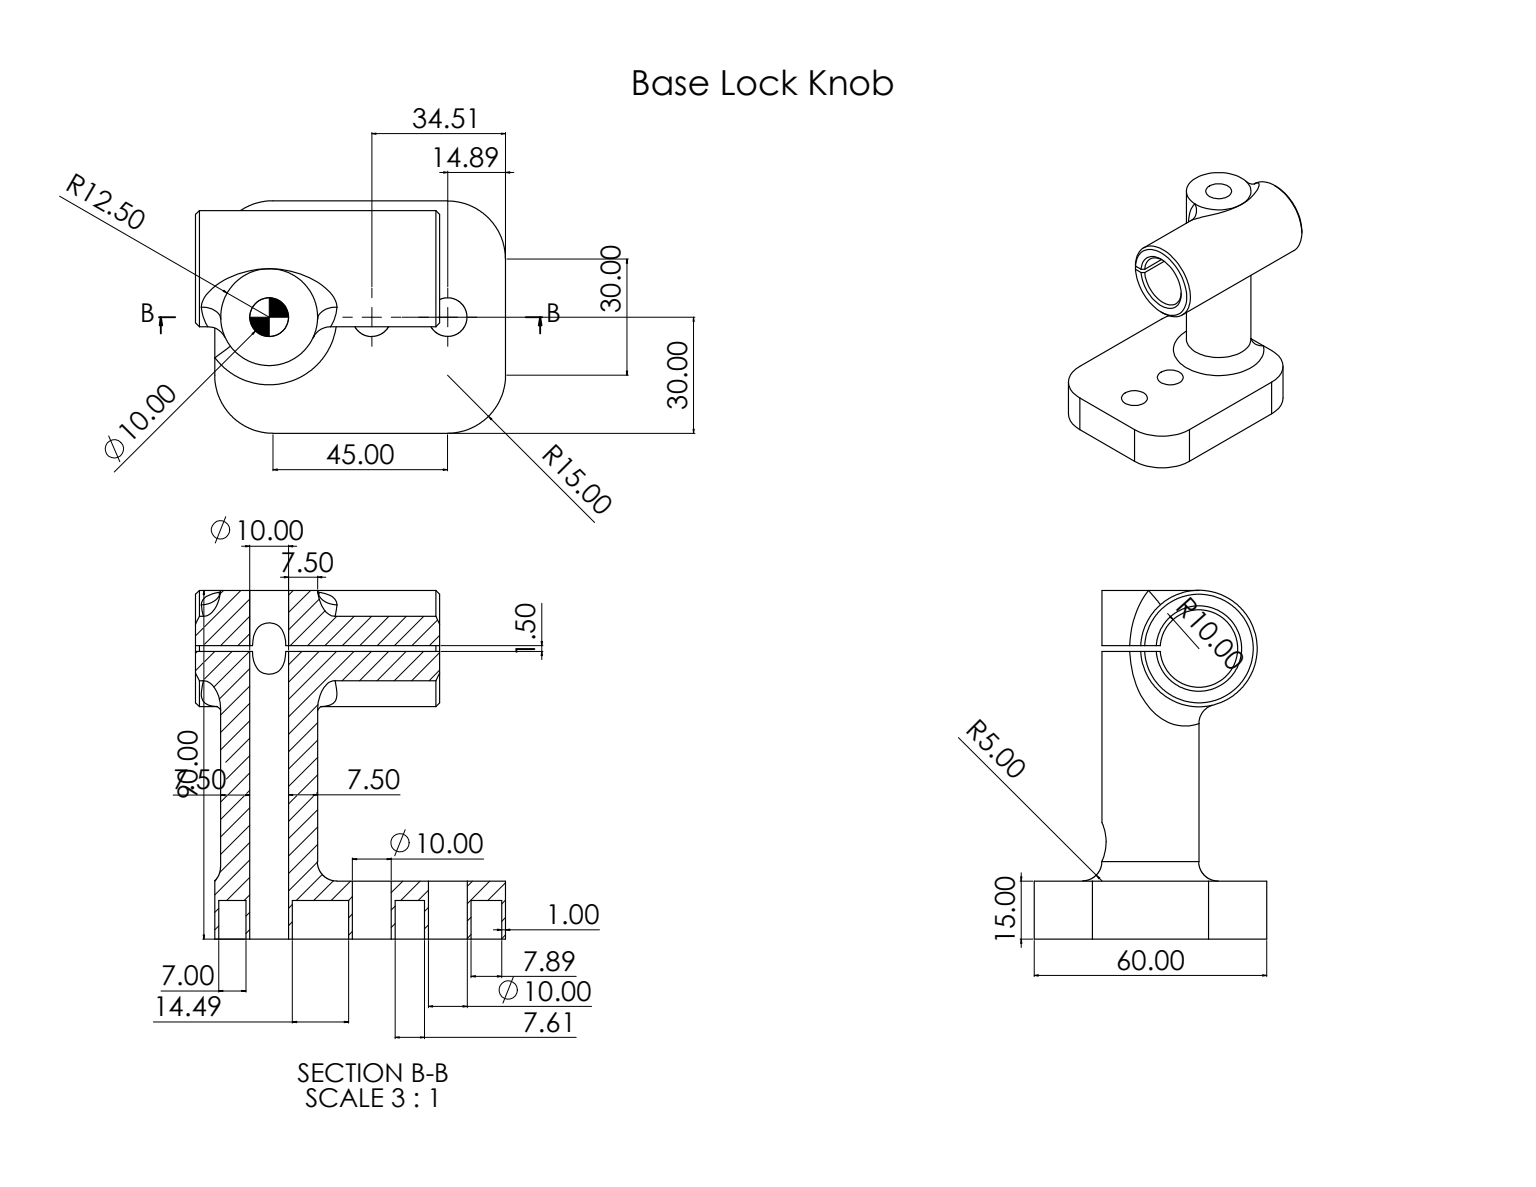
ISO-10303-21;
HEADER;
FILE_DESCRIPTION (('STEP AP214'),
    '1' );
FILE_NAME ('Base Lock Knob.step',
    '2026-10-26T22:46:44',
    ( '' ),
    ( '' ),
    'SwSTEP 2.0',
    'SolidWorks 2025',
    '' );
FILE_SCHEMA (( 'AUTOMOTIVE_DESIGN' ));
ENDSEC;

DATA;
#13=EDGE_CURVE ( 'NONE', #4124, #14697, #820, .T. ) ;
#15=CARTESIAN_POINT ( 'NONE',  ( -25.96080279087190945, 79.85293219504170281, -10.39653350028737755 ) ) ;
#19=CARTESIAN_POINT ( 'NONE',  ( 0.000000000000000000, -10.00000000000000000, 0.000000000000000000 ) ) ;
#40=CARTESIAN_POINT ( 'NONE',  ( -32.23733050826358237, 69.70612202061964524, 1.777571403100950187 ) ) ;
#44=CARTESIAN_POINT ( 'NONE',  ( -28.41953442586123302, 80.00000000005270806, -1.424835221693572684 ) ) ;
#49=AXIS2_PLACEMENT_3D ( 'NONE', #5119, #19642, #8405 ) ;
#53=ORIENTED_EDGE ( 'NONE', *, *, #309, .F. ) ;
#62=LINE ( 'NONE', #1856, #5490 ) ;
#65=CIRCLE ( 'NONE', #5111, 12.50000000000000000 ) ;
#69=CARTESIAN_POINT ( 'NONE',  ( -27.55705705607979894, 6.378909713838078588, -4.810857297669037358 ) ) ;
#72=ADVANCED_FACE ( 'NONE', ( #4104, #6856 ), #20110, .T. ) ;
#74=CARTESIAN_POINT ( 'NONE',  ( -3.712242387446013758, 47.26449505096422854, -2.316332963494041497 ) ) ;
#75=AXIS2_PLACEMENT_3D ( 'NONE', #8179, #20707, #4902 ) ;
#78=CARTESIAN_POINT ( 'NONE',  ( -4.898149591010308335, 50.01850704181430984, -13.27720951148779349 ) ) ;
#82=EDGE_CURVE ( 'NONE', #14650, #1521, #9980, .T. ) ;
#90=FACE_OUTER_BOUND ( 'NONE', #11303, .T. ) ;
#94=CARTESIAN_POINT ( 'NONE',  ( -20.20766917169448007, 62.83385617594171180, -2.712160011935111914 ) ) ;
#97=CARTESIAN_POINT ( 'NONE',  ( -14.59739189792666281, 58.60404727593866170, -4.812026853405405369 ) ) ;
#107=CARTESIAN_POINT ( 'NONE',  ( -32.72405129661866141, 57.94895811088655080, 0.7443064298479508123 ) ) ;
#126=CARTESIAN_POINT ( 'NONE',  ( -0.1767699604045824824, 64.25000000000000000, 2.481238266578627449 ) ) ;
#133=DIRECTION ( 'NONE',  ( -0.000000000000000000, 1.000000000000000000, -0.000000000000000000 ) ) ;
#143=CARTESIAN_POINT ( 'NONE',  ( -31.87136685185827645, 66.76123571212177410, 2.404802591979305237 ) ) ;
#151=CARTESIAN_POINT ( 'NONE',  ( -28.39898833977742854, 64.25000000000000000, 3.829121630900767848 ) ) ;
#162=EDGE_CURVE ( 'NONE', #4703, #13744, #13389, .T. ) ;
#166=VERTEX_POINT ( 'NONE', #7371 ) ;
#168=CARTESIAN_POINT ( 'NONE',  ( -15.61408887313298166, 45.63508326896292289, -12.50000000000000533 ) ) ;
#173=CARTESIAN_POINT ( 'NONE',  ( 0.8637328751229490509, 57.32143202600091314, 0.4056442452730588677 ) ) ;
#174=CARTESIAN_POINT ( 'NONE',  ( 0.2936549083987780584, 78.35468191082874512, -5.667085693055155637 ) ) ;
#180=ORIENTED_EDGE ( 'NONE', *, *, #8626, .T. ) ;
#196=VECTOR ( 'NONE', #4579, 1000.000000000000000 ) ;
#201=CARTESIAN_POINT ( 'NONE',  ( -32.31535884961043337, 59.90787884595005863, 1.627344972937480483 ) ) ;
#223=CYLINDRICAL_SURFACE ( 'NONE', #8286, 5.000000000000000000 ) ;
#228=EDGE_LOOP ( 'NONE', ( #1966, #14551, #9394, #914, #2067, #12471, #14821, #17580, #5403, #1919 ) ) ;
#245=VERTEX_POINT ( 'NONE', #13977 ) ;
#253=AXIS2_PLACEMENT_3D ( 'NONE', #1126, #2508, #8850 ) ;
#262=VECTOR ( 'NONE', #1217, 1000.000000000000000 ) ;
#269=CARTESIAN_POINT ( 'NONE',  ( -4.599716269004222369, 61.16723911170964811, 5.137000474222295665 ) ) ;
#273=CARTESIAN_POINT ( 'NONE',  ( 1.235636163673195176, 55.55531401624686794, -0.8411524222362073422 ) ) ;
#274=CARTESIAN_POINT ( 'NONE',  ( -27.29860958162435480, 65.74999999999997158, 5.347094680480812379 ) ) ;
#278=CARTESIAN_POINT ( 'NONE',  ( -28.99999999999999289, 0.000000000000000000, 15.00000000000000178 ) ) ;
#285=FACE_OUTER_BOUND ( 'NONE', #6570, .T. ) ;
#287=EDGE_LOOP ( 'NONE', ( #14816, #1290 ) ) ;
#301=CARTESIAN_POINT ( 'NONE',  ( -33.51155206502836137, 53.04833639938227208, -3.407080289749979229 ) ) ;
#309=EDGE_CURVE ( 'NONE', #20070, #6727, #13759, .T. ) ;
#324=EDGE_CURVE ( 'NONE', #1328, #16503, #11374, .T. ) ;
#329=AXIS2_PLACEMENT_3D ( 'NONE', #7780, #14388, #14489 ) ;
#336=PLANE ( 'NONE',  #16281 ) ;
#345=ORIENTED_EDGE ( 'NONE', *, *, #6765, .T. ) ;
#347=ORIENTED_EDGE ( 'NONE', *, *, #464, .T. ) ;
#348=ADVANCED_FACE ( 'NONE', ( #1860 ), #11088, .F. ) ;
#353=ORIENTED_EDGE ( 'NONE', *, *, #18968, .F. ) ;
#355=CARTESIAN_POINT ( 'NONE',  ( -21.06087829250213161, 79.98244021547201044, -11.72107194671396790 ) ) ;
#358=EDGE_CURVE ( 'NONE', #6609, #4749, #6287, .T. ) ;
#368=DIRECTION ( 'NONE',  ( -0.000000000000000000, -1.000000000000000000, -0.000000000000000000 ) ) ;
#369=EDGE_CURVE ( 'NONE', #14650, #14697, #6503, .T. ) ;
#372=FACE_OUTER_BOUND ( 'NONE', #9443, .T. ) ;
#373=CARTESIAN_POINT ( 'NONE',  ( -4.811817756148304426, 79.75568800831774752, -9.793444445058595349 ) ) ;
#387=CARTESIAN_POINT ( 'NONE',  ( -3.556084784758247075, 50.96167829366792290, 1.269699694002965007 ) ) ;
#388=CARTESIAN_POINT ( 'NONE',  ( -9.537558382401318369, 79.97813440949151698, -11.66361662172994507 ) ) ;
#396=ORIENTED_EDGE ( 'NONE', *, *, #17876, .T. ) ;
#407=CIRCLE ( 'NONE', #12256, 5.999999999999989342 ) ;
#408=DIRECTION ( 'NONE',  ( -1.000000000000000000, 0.000000000000000000, 0.000000000000000000 ) ) ;
#409=CARTESIAN_POINT ( 'NONE',  ( -15.99999999999999289, 80.00000000000000000, 0.000000000000000000 ) ) ;
#417=CARTESIAN_POINT ( 'NONE',  ( -33.37417213237042546, 54.75746433087826404, -1.535552296325748189 ) ) ;
#422=EDGE_CURVE ( 'NONE', #16527, #15321, #7895, .T. ) ;
#434=( BOUNDED_CURVE ( )  B_SPLINE_CURVE ( 3, ( #6259, #9555, #12753, #12546 ),
 .UNSPECIFIED., .F., .T. ) 
 B_SPLINE_CURVE_WITH_KNOTS ( ( 4, 4 ),
 ( 4.913746901175024107, 6.283185307179586232 ),
 .UNSPECIFIED. ) 
 CURVE ( )  GEOMETRIC_REPRESENTATION_ITEM ( )  RATIONAL_B_SPLINE_CURVE ( ( 1.000000000000000000, 0.8497311128276563430, 0.8497311128276563430, 1.000000000000000000 ) ) 
 REPRESENTATION_ITEM ( '' )  );
#448=ORIENTED_EDGE ( 'NONE', *, *, #2524, .T. ) ;
#461=CARTESIAN_POINT ( 'NONE',  ( -17.30116400286886247, 79.99994664032418257, -12.45114708371502665 ) ) ;
#463=CARTESIAN_POINT ( 'NONE',  ( 30.00000000000000355, 5.000000000000000000, 30.00000000000000000 ) ) ;
#464=EDGE_CURVE ( 'NONE', #15321, #2307, #18152, .T. ) ;
#476=CARTESIAN_POINT ( 'NONE',  ( -0.1767699604045824824, 64.25000000000000000, 2.481238266578627449 ) ) ;
#477=CARTESIAN_POINT ( 'NONE',  ( -3.836698435374707561, 79.99999999983937471, -2.903060217168568435 ) ) ;
#482=LINE ( 'NONE', #19857, #18341 ) ;
#487=CARTESIAN_POINT ( 'NONE',  ( -26.66796757275972851, 5.894401750582999533, 6.542839447999508451 ) ) ;
#491=VERTEX_POINT ( 'NONE', #4071 ) ;
#493=CARTESIAN_POINT ( 'NONE',  ( -3.931445803941664430, 46.62695496839331355, -3.273709564003291383 ) ) ;
#496=CARTESIAN_POINT ( 'NONE',  ( 0.5172280101801079999, 58.91385993483535799, 1.214474307743183434 ) ) ;
#497=CARTESIAN_POINT ( 'NONE',  ( 0.4210663660453498047, 78.26446952993892126, -5.493235020936472424 ) ) ;
#501=DIRECTION ( 'NONE',  ( -0.000000000000000000, -1.000000000000000000, -0.000000000000000000 ) ) ;
#520=CARTESIAN_POINT ( 'NONE',  ( -32.92944801084382078, 57.01857061577523922, 0.2052755498065614581 ) ) ;
#532=DIRECTION ( 'NONE',  ( -0.000000000000000000, 1.000000000000000000, -0.000000000000000000 ) ) ;
#533=AXIS2_PLACEMENT_3D ( 'NONE', #6159, #10536, #10317 ) ;
#541=CARTESIAN_POINT ( 'NONE',  ( 30.10683012259193703, 0.000000000000000000, 0.000000000000000000 ) ) ;
#553=( BOUNDED_CURVE ( )  B_SPLINE_CURVE ( 3, ( #9239, #19121, #12236, #18698 ),
 .UNSPECIFIED., .F., .F. ) 
 B_SPLINE_CURVE_WITH_KNOTS ( ( 4, 4 ),
 ( 0.000000000000000000, 1.369438406004562347 ),
 .UNSPECIFIED. ) 
 CURVE ( )  GEOMETRIC_REPRESENTATION_ITEM ( )  RATIONAL_B_SPLINE_CURVE ( ( 1.000000000000000000, 0.8497311128276563430, 0.8497311128276563430, 1.000000000000000000 ) ) 
 REPRESENTATION_ITEM ( '' )  );
#554=ORIENTED_EDGE ( 'NONE', *, *, #4724, .T. ) ;
#563=CARTESIAN_POINT ( 'NONE',  ( -26.10629707152433809, 79.63451458383349291, -9.058872303758411348 ) ) ;
#569=CARTESIAN_POINT ( 'NONE',  ( -30.20545447418457385, 64.25000000000001421, 2.744335235139487406 ) ) ;
#575=CARTESIAN_POINT ( 'NONE',  ( -2.600405991085453561, 77.88264414865945184, -4.670285688179051320 ) ) ;
#577=ORIENTED_EDGE ( 'NONE', *, *, #4172, .T. ) ;
#580=DIRECTION ( 'NONE',  ( 1.000000000000000000, 0.000000000000000000, 0.000000000000000000 ) ) ;
#583=EDGE_CURVE ( 'NONE', #14019, #631, #10846, .T. ) ;
#585=CARTESIAN_POINT ( 'NONE',  ( -29.99999999999999645, 5.000000000000000000, 9.729160503328165177 ) ) ;
#595=CARTESIAN_POINT ( 'NONE',  ( -3.729411824114762020, 52.78418889159976857, -3.786816875109808578 ) ) ;
#598=DIRECTION ( 'NONE',  ( -1.000000000000000000, -0.000000000000000000, -0.000000000000000000 ) ) ;
#603=CARTESIAN_POINT ( 'NONE',  ( 27.66662763442663220, 64.25000000000000000, -1.859747928060467181 ) ) ;
#615=CARTESIAN_POINT ( 'NONE',  ( -19.02430517209115735, 70.26110273505831572, -3.991204510516646931 ) ) ;
#616=EDGE_CURVE ( 'NONE', #631, #3306, #11174, .T. ) ;
#618=EDGE_CURVE ( 'NONE', #9039, #9755, #2936, .T. ) ;
#621=CARTESIAN_POINT ( 'NONE',  ( -28.23075158081314484, 53.16826294859335889, 2.609184450367471708 ) ) ;
#626=ORIENTED_EDGE ( 'NONE', *, *, #616, .T. ) ;
#631=VERTEX_POINT ( 'NONE', #3318 ) ;
#639=CARTESIAN_POINT ( 'NONE',  ( 30.00000000000000355, 5.000000000000000000, -15.00000000000000000 ) ) ;
#653=ORIENTED_EDGE ( 'NONE', *, *, #12072, .F. ) ;
#655=CARTESIAN_POINT ( 'NONE',  ( -14.99999999999999645, 0.000000000000000000, -15.00000000000000000 ) ) ;
#659=EDGE_LOOP ( 'NONE', ( #1271, #18731 ) ) ;
#661=CARTESIAN_POINT ( 'NONE',  ( -17.30014261508840434, 80.00000000000054001, -12.43489149392628512 ) ) ;
#662=FACE_OUTER_BOUND ( 'NONE', #2324, .T. ) ;
#664=ORIENTED_EDGE ( 'NONE', *, *, #14243, .F. ) ;
#675=EDGE_CURVE ( 'NONE', #11638, #6609, #8654, .T. ) ;
#681=VERTEX_POINT ( 'NONE', #19127 ) ;
#682=DIRECTION ( 'NONE',  ( -0.000000000000000000, 1.000000000000000000, -0.000000000000000000 ) ) ;
#686=DIRECTION ( 'NONE',  ( -1.000000000000000000, -0.000000000000000000, -0.000000000000000000 ) ) ;
#693=VECTOR ( 'NONE', #17106, 1000.000000000000000 ) ;
#702=EDGE_CURVE ( 'NONE', #19907, #9631, #6632, .T. ) ;
#710=CIRCLE ( 'NONE', #14277, 13.99999999999999822 ) ;
#711=EDGE_LOOP ( 'NONE', ( #17334, #865, #11449, #20358 ) ) ;
#714=CARTESIAN_POINT ( 'NONE',  ( 30.00000000000000355, 0.000000000000000000, -15.00000000000000000 ) ) ;
#720=DIRECTION ( 'NONE',  ( 0.000000000000000000, 0.000000000000000000, -1.000000000000000000 ) ) ;
#725=CYLINDRICAL_SURFACE ( 'NONE', #12270, 12.50000000000000000 ) ;
#726=CARTESIAN_POINT ( 'NONE',  ( -15.04600911323590218, 50.47255456144257835, -16.23554317993713170 ) ) ;
#737=ORIENTED_EDGE ( 'NONE', *, *, #2963, .F. ) ;
#739=DIRECTION ( 'NONE',  ( -0.000000000000000000, -0.000000000000000000, 1.000000000000000000 ) ) ;
#745=ORIENTED_EDGE ( 'NONE', *, *, #358, .F. ) ;
#752=DIRECTION ( 'NONE',  ( 0.000000000000000000, -0.000000000000000000, -1.000000000000000000 ) ) ;
#753=FACE_OUTER_BOUND ( 'NONE', #17256, .T. ) ;
#774=CARTESIAN_POINT ( 'NONE',  ( -16.26047902139016088, 79.99999999999998579, -12.49895143242785522 ) ) ;
#776=CARTESIAN_POINT ( 'NONE',  ( 30.00000000000000355, -10.00000000000000000, -28.99999999999999645 ) ) ;
#788=CARTESIAN_POINT ( 'NONE',  ( -15.47785876946503691, 80.00000332749893062, -12.49385289755957729 ) ) ;
#796=CARTESIAN_POINT ( 'NONE',  ( -28.50008649836227193, 6.470284334177582863, 0.3892821999670322275 ) ) ;
#801=AXIS2_PLACEMENT_3D ( 'NONE', #9097, #5597, #15294 ) ;
#810=ORIENTED_EDGE ( 'NONE', *, *, #11877, .F. ) ;
#819=CIRCLE ( 'NONE', #15126, 14.99999999999999645 ) ;
#820=LINE ( 'NONE', #20002, #17114 ) ;
#825=CARTESIAN_POINT ( 'NONE',  ( -10.99999999999999822, 15.09941697557068530, 0.9999999999999991118 ) ) ;
#826=DIRECTION ( 'NONE',  ( -0.000000000000000000, -0.000000000000000000, 1.000000000000000000 ) ) ;
#827=CARTESIAN_POINT ( 'NONE',  ( -17.49467092514650801, 49.50700362264424115, -12.43228238208896030 ) ) ;
#829=VECTOR ( 'NONE', #16903, 1000.000000000000000 ) ;
#851=CARTESIAN_POINT ( 'NONE',  ( -13.77465266732642846, 19.58876728727312511, 12.30409294039043466 ) ) ;
#854=CARTESIAN_POINT ( 'NONE',  ( -28.16307471351787228, 76.23982303504115521, 2.898234736985794591 ) ) ;
#865=ORIENTED_EDGE ( 'NONE', *, *, #17437, .F. ) ;
#868=EDGE_CURVE ( 'NONE', #1492, #2398, #16138, .T. ) ;
#876=CARTESIAN_POINT ( 'NONE',  ( -11.09376813494104397, 14.43059931244999028, 0.9644707416441876680 ) ) ;
#889=CARTESIAN_POINT ( 'NONE',  ( 30.10683012259193703, -24.14213562373095456, 0.000000000000000000 ) ) ;
#890=CARTESIAN_POINT ( 'NONE',  ( -15.47785959468120431, 80.00000000000014211, -12.49180211257053230 ) ) ;
#894=AXIS2_PLACEMENT_3D ( 'NONE', #1472, #17166, #19175 ) ;
#895=CARTESIAN_POINT ( 'NONE',  ( -12.69376962344485449, 11.33472108774821763, 12.05717403569970969 ) ) ;
#900=CARTESIAN_POINT ( 'NONE',  ( -28.22855330669906593, 8.912322265355541617, 2.677539729764461196 ) ) ;
#907=TOROIDAL_SURFACE ( 'NONE', #12088, 17.50000000000000000, 5.000000000000000000 ) ;
#914=ORIENTED_EDGE ( 'NONE', *, *, #14759, .T. ) ;
#916=LINE ( 'NONE', #12659, #16572 ) ;
#919=EDGE_CURVE ( 'NONE', #2330, #10554, #16387, .T. ) ;
#932=CARTESIAN_POINT ( 'NONE',  ( -14.62719308666609486, 45.60972712416246111, -12.42922832581293413 ) ) ;
#947=PLANE ( 'NONE',  #10845 ) ;
#948=CARTESIAN_POINT ( 'NONE',  ( -1.752364627967215149, 50.08700668601604633, -10.77852995906744304 ) ) ;
#949=LINE ( 'NONE', #17067, #3578 ) ;
#993=CARTESIAN_POINT ( 'NONE',  ( -4.579930894573177369, 68.94695149080686747, 5.083831496961729535 ) ) ;
#1002=CARTESIAN_POINT ( 'NONE',  ( -15.66959223257168432, 10.09941697557068707, 12.50000000000000000 ) ) ;
#1005=CARTESIAN_POINT ( 'NONE',  ( -26.38519111739858758, 79.82398913006802843, -10.19891841068203142 ) ) ;
#1007=CARTESIAN_POINT ( 'NONE',  ( -33.99999999999997868, 64.25000000000000000, -2.528164662410438357 ) ) ;
#1022=ORIENTED_EDGE ( 'NONE', *, *, #6255, .F. ) ;
#1034=AXIS2_PLACEMENT_3D ( 'NONE', #19639, #3534, #16472 ) ;
#1035=LINE ( 'NONE', #20422, #19941 ) ;
#1038=CARTESIAN_POINT ( 'NONE',  ( -13.06364034290321463, 49.50854601617997020, -12.17427138426762312 ) ) ;
#1050=VECTOR ( 'NONE', #11952, 1000.000000000000000 ) ;
#1054=CARTESIAN_POINT ( 'NONE',  ( -15.99999999999999289, 64.25000000000000000, 0.000000000000000000 ) ) ;
#1056=CARTESIAN_POINT ( 'NONE',  ( -31.72276537669240071, 50.43494788623335268, -8.899223764819897298 ) ) ;
#1057=CARTESIAN_POINT ( 'NONE',  ( 30.10683012259193703, -10.00000000000000000, 5.999999999999998224 ) ) ;
#1062=VECTOR ( 'NONE', #16123, 1000.000000000000000 ) ;
#1081=CARTESIAN_POINT ( 'NONE',  ( 0.2040382970959897513, 69.52210068921742447, 1.838693167884630109 ) ) ;
#1102=CARTESIAN_POINT ( 'NONE',  ( -15.99999999999999289, 0.000000000000000000, 0.000000000000000000 ) ) ;
#1105=CARTESIAN_POINT ( 'NONE',  ( -10.99999999999999822, 15.09941697557068530, 0.9999999999999991118 ) ) ;
#1107=LINE ( 'NONE', #7760, #18343 ) ;
#1108=CARTESIAN_POINT ( 'NONE',  ( -15.99999999999999289, 79.99999999999998579, -12.50000000000000000 ) ) ;
#1111=CARTESIAN_POINT ( 'NONE',  ( -14.85679855891570078, 10.22906252849420561, 12.44867321866860266 ) ) ;
#1120=CARTESIAN_POINT ( 'NONE',  ( -34.66668267600675080, 65.74999999999997158, 1.813692929321156555 ) ) ;
#1123=ORIENTED_EDGE ( 'NONE', *, *, #8792, .F. ) ;
#1126=CARTESIAN_POINT ( 'NONE',  ( -14.99999999999999645, 5.000000000000000000, -15.00000000000000000 ) ) ;
#1128=B_SPLINE_CURVE_WITH_KNOTS ( 'NONE', 3,
 ( #9917, #10017, #6633, #8123, #3363, #97, #8337, #16412, #19680, #1576, #5155, #2688, #13233, #6424, #3571, #11641, #3162, #18105, #4852, #11425 ),
 .UNSPECIFIED., .F., .F.,
 ( 4, 2, 2, 2, 2, 2, 2, 2, 2, 4 ),
 ( 0.008555345346386149588, 0.009089294358497906207, 0.009623243370609659356, 0.01069114139483316739, 0.01175903941905667716, 0.01282693744328018692, 0.01389483546750369669, 0.01496273349172720646, 0.01603063151595071623, 0.01709852954017422599 ),
 .UNSPECIFIED. ) ;
#1135=VERTEX_POINT ( 'NONE', #6351 ) ;
#1139=CARTESIAN_POINT ( 'NONE',  ( -20.49080202807238393, 12.87717145046493172, 11.66622392198317293 ) ) ;
#1150=CARTESIAN_POINT ( 'NONE',  ( -26.36906608345258363, 50.04675353776782742, -13.70410848631408385 ) ) ;
#1153=CARTESIAN_POINT ( 'NONE',  ( -28.15281455745353512, 46.83340527910446838, -2.943232864391990056 ) ) ;
#1160=CARTESIAN_POINT ( 'NONE',  ( -3.496475329869574100, 79.99999999992608934, -0.04629550956327706246 ) ) ;
#1165=CARTESIAN_POINT ( 'NONE',  ( 1.088894091976222667, 56.28116656631951997, -0.2880183321277288155 ) ) ;
#1166=CARTESIAN_POINT ( 'NONE',  ( -28.50046567980698242, 8.570075179949460775, 0.3245954035919153546 ) ) ;
#1172=FACE_OUTER_BOUND ( 'NONE', #8065, .T. ) ;
#1178=CARTESIAN_POINT ( 'NONE',  ( 26.99999999999999645, 65.00000000000000000, -12.50000000000000000 ) ) ;
#1193=FACE_OUTER_BOUND ( 'NONE', #1883, .T. ) ;
#1199=AXIS2_PLACEMENT_3D ( 'NONE', #15525, #15733, #4369 ) ;
#1212=CARTESIAN_POINT ( 'NONE',  ( -11.26027265087348894, 13.47399565661562626, 11.56734157159816156 ) ) ;
#1217=DIRECTION ( 'NONE',  ( -1.000000000000000000, -0.000000000000000000, -0.000000000000000000 ) ) ;
#1220=EDGE_LOOP ( 'NONE', ( #180, #19438, #20677, #16352, #3094, #19216, #16530, #18642, #15744, #18492, #577, #6988, #3840, #11038, #4651 ) ) ;
#1225=DIRECTION ( 'NONE',  ( 0.000000000000000000, 0.000000000000000000, -1.000000000000000000 ) ) ;
#1229=CARTESIAN_POINT ( 'NONE',  ( 10.49211908931699178, -24.14213562373095456, 0.000000000000000000 ) ) ;
#1245=ORIENTED_EDGE ( 'NONE', *, *, #4758, .T. ) ;
#1250=CARTESIAN_POINT ( 'NONE',  ( -11.24740156498038779, 50.36046179987343407, -15.77731508861108445 ) ) ;
#1254=CARTESIAN_POINT ( 'NONE',  ( -21.23833354872890311, 45.29156160041301860, -11.37540731453001541 ) ) ;
#1257=CARTESIAN_POINT ( 'NONE',  ( -15.99999999999999289, 15.09941697557068530, 0.9999999999999991118 ) ) ;
#1258=CARTESIAN_POINT ( 'NONE',  ( -25.99999999999999645, 9.999999999999994671, 7.500000000000000000 ) ) ;
#1263=FACE_OUTER_BOUND ( 'NONE', #4142, .T. ) ;
#1266=CARTESIAN_POINT ( 'NONE',  ( -31.04127923955400803, 50.23417253100409852, -9.842805686593695924 ) ) ;
#1269=ADVANCED_FACE ( 'NONE', ( #16339 ), #11667, .T. ) ;
#1271=ORIENTED_EDGE ( 'NONE', *, *, #5205, .T. ) ;
#1274=DIRECTION ( 'NONE',  ( 0.000000000000000000, 0.000000000000000000, 1.000000000000000000 ) ) ;
#1281=CARTESIAN_POINT ( 'NONE',  ( -27.88482465330859839, 73.88542888634933092, 3.878668165723263339 ) ) ;
#1282=CARTESIAN_POINT ( 'NONE',  ( -20.33207080104639530, 17.61692987535746369, 11.72687972142948709 ) ) ;
#1283=EDGE_CURVE ( 'NONE', #13189, #11638, #14723, .T. ) ;
#1285=CARTESIAN_POINT ( 'NONE',  ( -28.65129735818244683, 65.53858748455373018, 2.490407514064852723 ) ) ;
#1288=VERTEX_POINT ( 'NONE', #3599 ) ;
#1290=ORIENTED_EDGE ( 'NONE', *, *, #8492, .F. ) ;
#1292=CARTESIAN_POINT ( 'NONE',  ( 30.10683012259193703, -10.00000000000000000, -5.999999999999998224 ) ) ;
#1293=CARTESIAN_POINT ( 'NONE',  ( -14.99999999999999822, 0.000000000000000000, -28.99999999999999645 ) ) ;
#1303=DIRECTION ( 'NONE',  ( -0.000000000000000000, -1.000000000000000000, -0.000000000000000000 ) ) ;
#1318=CARTESIAN_POINT ( 'NONE',  ( -35.00000000000000000, 65.00000000000000000, -27.49999999999999645 ) ) ;
#1322=CIRCLE ( 'NONE', #9753, 15.00000000000000000 ) ;
#1328=VERTEX_POINT ( 'NONE', #16749 ) ;
#1332=DIRECTION ( 'NONE',  ( 0.000000000000000000, 0.000000000000000000, -1.000000000000000000 ) ) ;
#1352=CARTESIAN_POINT ( 'NONE',  ( -4.908256850829183726, 51.34256347499046313, -6.001213154916446690 ) ) ;
#1353=CARTESIAN_POINT ( 'NONE',  ( -15.99999999999999289, 5.000000000000000000, 0.000000000000000000 ) ) ;
#1362=EDGE_LOOP ( 'NONE', ( #19782, #2741, #18153, #20632 ) ) ;
#1367=CARTESIAN_POINT ( 'NONE',  ( -3.506621468774197670, 49.99927930435590184, -12.32165535527945721 ) ) ;
#1370=CIRCLE ( 'NONE', #10141, 5.999999999999998224 ) ;
#1372=DIRECTION ( 'NONE',  ( 0.000000000000000000, 0.000000000000000000, -1.000000000000000000 ) ) ;
#1373=ADVANCED_FACE ( 'NONE', ( #1172 ), #20136, .F. ) ;
#1380=AXIS2_PLACEMENT_3D ( 'NONE', #19536, #19849, #3737 ) ;
#1382=CARTESIAN_POINT ( 'NONE',  ( -29.99999999999999645, 5.000000000000000000, 10.50000000000000000 ) ) ;
#1383=VECTOR ( 'NONE', #9881, 1000.000000000000000 ) ;
#1388=VECTOR ( 'NONE', #2434, 1000.000000000000000 ) ;
#1391=EDGE_CURVE ( 'NONE', #6871, #9451, #11642, .T. ) ;
#1393=CARTESIAN_POINT ( 'NONE',  ( -4.294235668597638167, 72.30161019875538386, 4.406123080991324770 ) ) ;
#1396=CARTESIAN_POINT ( 'NONE',  ( -24.67152222510459580, 79.91873556435304238, -10.93282151138175173 ) ) ;
#1402=LINE ( 'NONE', #20781, #4685 ) ;
#1404=CARTESIAN_POINT ( 'NONE',  ( -15.99999999999999289, 80.00000000000000000, 4.999999999999989342 ) ) ;
#1420=CARTESIAN_POINT ( 'NONE',  ( -28.48686108716033516, 80.00000000007401013, -0.6469719004584603139 ) ) ;
#1421=VERTEX_POINT ( 'NONE', #14005 ) ;
#1429=CARTESIAN_POINT ( 'NONE',  ( -27.61765422622016430, 80.00000000021789504, -4.628091497302904145 ) ) ;
#1432=B_SPLINE_CURVE_WITH_KNOTS ( 'NONE', 3,
 ( #9831, #19482, #11027, #4963 ),
 .UNSPECIFIED., .F., .F.,
 ( 4, 4 ),
 ( 4.336808689942017736E-18, 0.001415162808320489293 ),
 .UNSPECIFIED. ) ;
#1440=VERTEX_POINT ( 'NONE', #10589 ) ;
#1457=CARTESIAN_POINT ( 'NONE',  ( -7.049456388680209074, 44.99877348914139930, -8.732428919826512370 ) ) ;
#1463=DIRECTION ( 'NONE',  ( 1.000000000000000000, 0.000000000000000000, 0.000000000000000000 ) ) ;
#1465=CARTESIAN_POINT ( 'NONE',  ( -11.00827370573233566, 79.99999999999128875, -11.47115151921867238 ) ) ;
#1472=CARTESIAN_POINT ( 'NONE',  ( 28.00000000000001066, 65.00000000000000000, -12.50000000000000000 ) ) ;
#1476=ADVANCED_FACE ( 'NONE', ( #8996, #20035 ), #12312, .T. ) ;
#1477=CARTESIAN_POINT ( 'NONE',  ( 0.2373305082636106289, 69.70612202061965945, 1.777571403100949743 ) ) ;
#1481=CARTESIAN_POINT ( 'NONE',  ( -35.00000000000000000, 65.00000000000000000, -12.50000000000000000 ) ) ;
#1483=CARTESIAN_POINT ( 'NONE',  ( -31.99680141974825531, 61.98207243580021242, 2.197686203131483662 ) ) ;
#1486=CARTESIAN_POINT ( 'NONE',  ( -27.32414976724623301, 67.00845937186198853, 5.293280639215754313 ) ) ;
#1487=CARTESIAN_POINT ( 'NONE',  ( -34.00000000000000711, 65.00000000000000000, -12.50000000000000000 ) ) ;
#1488=CARTESIAN_POINT ( 'NONE',  ( 27.00000000000002487, 64.25000000000000000, 2.481238266578627449 ) ) ;
#1492=VERTEX_POINT ( 'NONE', #20548 ) ;
#1494=CARTESIAN_POINT ( 'NONE',  ( -3.243958593759534104, 64.25000000000001421, 3.524958307384021161 ) ) ;
#1509=DIRECTION ( 'NONE',  ( -0.000000000000000000, -1.000000000000000000, -0.000000000000000000 ) ) ;
#1514=EDGE_LOOP ( 'NONE', ( #7636, #5356, #53, #5961 ) ) ;
#1521=VERTEX_POINT ( 'NONE', #13209 ) ;
#1528=B_SPLINE_CURVE_WITH_KNOTS ( 'NONE', 3,
 ( #2709, #15652, #1120, #7563 ),
 .UNSPECIFIED., .F., .F.,
 ( 4, 4 ),
 ( 0.000000000000000000, 0.001415162808320496448 ),
 .UNSPECIFIED. ) ;
#1530=EDGE_LOOP ( 'NONE', ( #1123, #6318, #16160, #7476, #6971, #5330, #6903, #19698 ) ) ;
#1549=FACE_OUTER_BOUND ( 'NONE', #4665, .T. ) ;
#1553=CARTESIAN_POINT ( 'NONE',  ( -30.00000000000017408, 4.999999999999888090, -5.972363130614329663 ) ) ;
#1556=ORIENTED_EDGE ( 'NONE', *, *, #17828, .F. ) ;
#1558=CARTESIAN_POINT ( 'NONE',  ( -9.459184262262997578, 45.14452168132807230, -10.67415978328379644 ) ) ;
#1561=DIRECTION ( 'NONE',  ( 1.000000000000000000, 0.000000000000000000, 0.000000000000000000 ) ) ;
#1568=CARTESIAN_POINT ( 'NONE',  ( -11.91377925401460303, 79.99311222855632764, -11.99929078098838353 ) ) ;
#1574=CARTESIAN_POINT ( 'NONE',  ( -31.96031196521626683, 62.29327126685349469, 2.258945850240144271 ) ) ;
#1576=CARTESIAN_POINT ( 'NONE',  ( -12.97569482790883910, 59.73889726494167007, -3.991204510516653148 ) ) ;
#1585=CARTESIAN_POINT ( 'NONE',  ( -32.44758470016270024, 59.24237906757368677, 1.369529638433351737 ) ) ;
#1598=CARTESIAN_POINT ( 'NONE',  ( -4.615602823079929529, 68.36083330499455712, 5.162430512331780186 ) ) ;
#1601=CARTESIAN_POINT ( 'NONE',  ( -28.42834865230874541, 79.61890673690945164, -9.096465090019584920 ) ) ;
#1605=AXIS2_PLACEMENT_3D ( 'NONE', #3807, #5810, #8684 ) ;
#1613=CARTESIAN_POINT ( 'NONE',  ( 30.00000000000000355, 5.000000000000000000, -30.00000000000000000 ) ) ;
#1625=ORIENTED_EDGE ( 'NONE', *, *, #82, .F. ) ;
#1627=CARTESIAN_POINT ( 'NONE',  ( -31.82323003959540486, 65.74999999999997158, 2.481238266578629226 ) ) ;
#1630=CARTESIAN_POINT ( 'NONE',  ( -28.40027614393203237, 79.99999999992436983, -1.584264587336083219 ) ) ;
#1639=LINE ( 'NONE', #12681, #3977 ) ;
#1653=CARTESIAN_POINT ( 'NONE',  ( -28.14076360089397610, 6.485357845765030937, -3.101869372784200163 ) ) ;
#1655=EDGE_CURVE ( 'NONE', #9209, #8656, #18501, .T. ) ;
#1662=CARTESIAN_POINT ( 'NONE',  ( -10.67320097367628051, 45.27968546322713195, -11.31348108637220484 ) ) ;
#1668=ORIENTED_EDGE ( 'NONE', *, *, #868, .T. ) ;
#1673=CARTESIAN_POINT ( 'NONE',  ( -1.754678344426114700, 79.23832348577455775, -7.772177369786309242 ) ) ;
#1675=DIRECTION ( 'NONE',  ( 0.000000000000000000, 0.000000000000000000, -1.000000000000000000 ) ) ;
#1677=CARTESIAN_POINT ( 'NONE',  ( -32.65293543921481501, 58.27329718154535954, 0.9126919759745467653 ) ) ;
#1679=ORIENTED_EDGE ( 'NONE', *, *, #12719, .T. ) ;
#1687=CARTESIAN_POINT ( 'NONE',  ( -28.78142635522318926, 60.56397566246508291, 1.839220826256013464 ) ) ;
#1688=CARTESIAN_POINT ( 'NONE',  ( -20.95922626054125004, 15.75780479222803265, 11.47416194257517041 ) ) ;
#1693=AXIS2_PLACEMENT_3D ( 'NONE', #6289, #4611, #1332 ) ;
#1699=ORIENTED_EDGE ( 'NONE', *, *, #3301, .F. ) ;
#1708=AXIS2_PLACEMENT_3D ( 'NONE', #1229, #4300, #7575 ) ;
#1716=ORIENTED_EDGE ( 'NONE', *, *, #369, .F. ) ;
#1718=CIRCLE ( 'NONE', #9476, 15.00000000000000000 ) ;
#1723=CARTESIAN_POINT ( 'NONE',  ( -15.63739925482664539, 71.60309586965422568, -4.990008254056941261 ) ) ;
#1729=DIRECTION ( 'NONE',  ( -1.000000000000000000, 0.000000000000000000, 0.000000000000000000 ) ) ;
#1737=AXIS2_PLACEMENT_3D ( 'NONE', #6501, #8089, #4719 ) ;
#1743=CARTESIAN_POINT ( 'NONE',  ( -29.34689839943911238, 64.25000000000000000, 3.131020379152387623 ) ) ;
#1747=CYLINDRICAL_SURFACE ( 'NONE', #20698, 15.00000000000000000 ) ;
#1758=DIRECTION ( 'NONE',  ( 0.000000000000000000, -1.000000000000000000, 0.000000000000000000 ) ) ;
#1763=CARTESIAN_POINT ( 'NONE',  ( -4.337715088898757898, 58.14881678702032985, 4.504901070458046775 ) ) ;
#1768=CARTESIAN_POINT ( 'NONE',  ( -3.348706032858273396, 64.03431171952128409, 2.490437087486337298 ) ) ;
#1769=LINE ( 'NONE', #6618, #14371 ) ;
#1770=CIRCLE ( 'NONE', #13629, 15.00000000000000000 ) ;
#1779=CARTESIAN_POINT ( 'NONE',  ( 28.00000000000001066, 65.00000000000000000, -12.50000000000000000 ) ) ;
#1783=CARTESIAN_POINT ( 'NONE',  ( -19.90328892528527405, 61.49158825347216606, -3.129485610713140353 ) ) ;
#1785=CARTESIAN_POINT ( 'NONE',  ( -33.26897445441569801, 55.37895663941098690, -0.9854948372298418802 ) ) ;
#1793=CIRCLE ( 'NONE', #16349, 5.000000000000000000 ) ;
#1798=CARTESIAN_POINT ( 'NONE',  ( -27.29420858402278682, 64.79389399373982883, 5.356384271183856960 ) ) ;
#1810=CARTESIAN_POINT ( 'NONE',  ( -27.50181195973150494, 65.74999999999997158, 4.917720511238727887 ) ) ;
#1813=AXIS2_PLACEMENT_3D ( 'NONE', #9999, #7543, #10724 ) ;
#1814=CARTESIAN_POINT ( 'NONE',  ( 10.49211908931699178, -24.14213562373095456, 0.000000000000000000 ) ) ;
#1823=CYLINDRICAL_SURFACE ( 'NONE', #6787, 4.999999999999989342 ) ;
#1833=EDGE_LOOP ( 'NONE', ( #10105, #17446, #8430, #4713 ) ) ;
#1840=CARTESIAN_POINT ( 'NONE',  ( -29.39959400891148533, 77.88264414865577123, -4.670285688177608918 ) ) ;
#1856=CARTESIAN_POINT ( 'NONE',  ( -34.00000000000000711, 65.00000000000000000, -27.49999999999999645 ) ) ;
#1860=FACE_OUTER_BOUND ( 'NONE', #8789, .T. ) ;
#1861=CARTESIAN_POINT ( 'NONE',  ( -26.51210826115306318, 5.754273642521425813, -6.783243196509797457 ) ) ;
#1866=CARTESIAN_POINT ( 'NONE',  ( -3.498163565539533337, 49.91419972531922156, 0.4740846950075849331 ) ) ;
#1870=CARTESIAN_POINT ( 'NONE',  ( -4.083084354063197807, 52.23701737708404380, -4.580011168034334723 ) ) ;
#1883=EDGE_LOOP ( 'NONE', ( #3229, #4307, #19456, #15845, #18900, #20146, #15930, #6724 ) ) ;
#1884=CARTESIAN_POINT ( 'NONE',  ( -16.36260074517335283, 58.39690413034580274, -4.990008254056941261 ) ) ;
#1893=VERTEX_POINT ( 'NONE', #20396 ) ;
#1898=CARTESIAN_POINT ( 'NONE',  ( -28.34314883718211320, 47.50472042562527974, -1.997976258590732357 ) ) ;
#1914=EDGE_CURVE ( 'NONE', #8547, #166, #1528, .T. ) ;
#1919=ORIENTED_EDGE ( 'NONE', *, *, #12734, .T. ) ;
#1935=CARTESIAN_POINT ( 'NONE',  ( -15.99999999999999289, 0.000000000000000000, -5.999999999999989342 ) ) ;
#1944=CARTESIAN_POINT ( 'NONE',  ( -21.12997896807823039, 79.99099046118983836, -11.97147087692114908 ) ) ;
#1947=EDGE_LOOP ( 'NONE', ( #10928, #1716, #4017, #6775 ) ) ;
#1949=CARTESIAN_POINT ( 'NONE',  ( -35.00000000000000000, 65.74999999999997158, 2.481238266578629226 ) ) ;
#1964=CARTESIAN_POINT ( 'NONE',  ( -28.22702101948337727, 8.914004613553291989, -2.683272181370100373 ) ) ;
#1966=ORIENTED_EDGE ( 'NONE', *, *, #13190, .F. ) ;
#1970=CARTESIAN_POINT ( 'NONE',  ( -15.99999999999998934, 45.63508326896292289, -12.50000000000000000 ) ) ;
#1971=ORIENTED_EDGE ( 'NONE', *, *, #2660, .T. ) ;
#1973=CARTESIAN_POINT ( 'NONE',  ( 1.058706124573915330, 56.42280402523184080, -0.1889998745171357630 ) ) ;
#1974=CARTESIAN_POINT ( 'NONE',  ( -13.67010713483751694, 79.99972648321134727, -12.39549370732874500 ) ) ;
#1983=CARTESIAN_POINT ( 'NONE',  ( -15.99999999999999289, 15.09941697557068530, 0.9999999999999991118 ) ) ;
#1989=FACE_OUTER_BOUND ( 'NONE', #12300, .T. ) ;
#2001=CARTESIAN_POINT ( 'NONE',  ( -27.72914186237699852, 52.00221496603906246, -4.940454205004202848 ) ) ;
#2002=CARTESIAN_POINT ( 'NONE',  ( -19.05461073270698336, 19.07106427949856808, 12.12416053983767839 ) ) ;
#2006=B_SPLINE_CURVE_WITH_KNOTS ( 'NONE', 3,
 ( #16785, #2691, #7332, #2264 ),
 .UNSPECIFIED., .F., .F.,
 ( 4, 4 ),
 ( 0.002660042459396035584, 0.003652875122883113713 ),
 .UNSPECIFIED. ) ;
#2007=EDGE_LOOP ( 'NONE', ( #18438, #3617, #11366, #18798 ) ) ;
#2009=EDGE_LOOP ( 'NONE', ( #17589, #3058, #9743, #1679, #9388 ) ) ;
#2013=CARTESIAN_POINT ( 'NONE',  ( -15.99999999999999289, -10.00000000000000000, 0.000000000000000000 ) ) ;
#2022=CARTESIAN_POINT ( 'NONE',  ( -15.99999999999999289, 80.00000000000000000, 4.999999999999989342 ) ) ;
#2026=B_SPLINE_CURVE_WITH_KNOTS ( 'NONE', 3,
 ( #5554, #4087, #8952, #10324 ),
 .UNSPECIFIED., .F., .F.,
 ( 4, 4 ),
 ( 2.602085213965210642E-18, 0.001415162808320503387 ),
 .UNSPECIFIED. ) ;
#2049=CARTESIAN_POINT ( 'NONE',  ( -16.26048281100938553, 80.00000000000179057, -12.49947570859690593 ) ) ;
#2060=CARTESIAN_POINT ( 'NONE',  ( -34.00000000000000711, 65.74999999999997158, 2.481238266578629226 ) ) ;
#2062=EDGE_LOOP ( 'NONE', ( #17293, #12292 ) ) ;
#2063=CARTESIAN_POINT ( 'NONE',  ( -27.29860958162435480, 64.25000000000000000, 5.347094680480811490 ) ) ;
#2064=CARTESIAN_POINT ( 'NONE',  ( -14.69883599711670286, 79.99994663880958967, -12.45114708389669467 ) ) ;
#2067=ORIENTED_EDGE ( 'NONE', *, *, #8234, .T. ) ;
#2075=CONICAL_SURFACE ( 'NONE', #16626, 11.00000000000001066, 0.7853981633974439491 ) ;
#2077=ORIENTED_EDGE ( 'NONE', *, *, #15147, .F. ) ;
#2082=CARTESIAN_POINT ( 'NONE',  ( 27.33334827330880756, 64.25000000000000000, 2.147472525011946409 ) ) ;
#2083=CARTESIAN_POINT ( 'NONE',  ( -3.106223272040122385, 58.44026525808256878, 1.004519969053611961 ) ) ;
#2092=ORIENTED_EDGE ( 'NONE', *, *, #2963, .T. ) ;
#2093=CARTESIAN_POINT ( 'NONE',  ( -18.48100260771138537, 10.09941697557069595, 4.999999999999990230 ) ) ;
#2096=CIRCLE ( 'NONE', #14645, 13.99999999999998757 ) ;
#2113=CARTESIAN_POINT ( 'NONE',  ( -27.31833330065622434, 51.55613243686521940, -5.649883545827639075 ) ) ;
#2133=LINE ( 'NONE', #2022, #12853 ) ;
#2135=DIRECTION ( 'NONE',  ( 1.000000000000000000, 0.000000000000000000, 0.000000000000000000 ) ) ;
#2140=DIRECTION ( 'NONE',  ( -1.000000000000000000, -0.000000000000000000, -0.000000000000000000 ) ) ;
#2146=CARTESIAN_POINT ( 'NONE',  ( -14.77002974211693953, 71.43993639942684126, -4.849479976237960344 ) ) ;
#2153=EDGE_CURVE ( 'NONE', #3073, #7189, #13609, .T. ) ;
#2163=CARTESIAN_POINT ( 'NONE',  ( -31.82323003959540486, 64.25000000000000000, 2.481238266578627449 ) ) ;
#2170=CARTESIAN_POINT ( 'NONE',  ( -1.416671275182913803, 79.14063577707194952, -7.486051927416997209 ) ) ;
#2175=DIRECTION ( 'NONE',  ( 0.000000000000000000, 0.000000000000000000, 1.000000000000000000 ) ) ;
#2180=CARTESIAN_POINT ( 'NONE',  ( -26.51357854883240250, 5.755818230185494322, 6.781050089207113274 ) ) ;
#2185=CARTESIAN_POINT ( 'NONE',  ( -14.45130347081977895, 45.60283267264664175, -12.40976118032397579 ) ) ;
#2188=CARTESIAN_POINT ( 'NONE',  ( 1.337262051077171554, 52.04110715870329074, -4.937170952670085100 ) ) ;
#2189=CARTESIAN_POINT ( 'NONE',  ( 0.7730453538337805908, 77.96698928858462807, -4.956659039178682669 ) ) ;
#2202=CARTESIAN_POINT ( 'NONE',  ( 30.10683012259193703, -10.00000000000000000, 0.000000000000000000 ) ) ;
#2203=DIRECTION ( 'NONE',  ( 0.000000000000000000, 1.000000000000000000, 0.000000000000000000 ) ) ;
#2206=CARTESIAN_POINT ( 'NONE',  ( -19.54313540116165271, 69.44160316133660160, -3.534893197518165664 ) ) ;
#2212=CARTESIAN_POINT ( 'NONE',  ( -26.24293131821966440, 50.67981595510417492, -7.209414086732143900 ) ) ;
#2233=DIRECTION ( 'NONE',  ( -0.000000000000000000, 1.000000000000000000, -0.000000000000000000 ) ) ;
#2240=CARTESIAN_POINT ( 'NONE',  ( -28.91711977134676204, 72.10661837392655116, 0.7232648427664161161 ) ) ;
#2242=CARTESIAN_POINT ( 'NONE',  ( 10.49211908931699178, -24.14213562373095456, 5.000000000000000000 ) ) ;
#2245=VECTOR ( 'NONE', #4734, 1000.000000000000000 ) ;
#2254=EDGE_LOOP ( 'NONE', ( #10674, #19755, #8751, #5116, #17485 ) ) ;
#2256=CARTESIAN_POINT ( 'NONE',  ( -18.07811133437977347, 79.99981534483862333, -12.41883285859719344 ) ) ;
#2264=CARTESIAN_POINT ( 'NONE',  ( -11.10102051443364779, 16.09941697557071905, 0.9999999999999997780 ) ) ;
#2270=CARTESIAN_POINT ( 'NONE',  ( -14.95778962878673823, 79.99997668367075221, -12.46941917154138579 ) ) ;
#2271=VERTEX_POINT ( 'NONE', #17200 ) ;
#2279=DIRECTION ( 'NONE',  ( 0.000000000000000000, 0.000000000000000000, -1.000000000000000000 ) ) ;
#2280=CARTESIAN_POINT ( 'NONE',  ( -27.39280497843907369, 9.626916829668232367, 5.187444349353440565 ) ) ;
#2289=CARTESIAN_POINT ( 'NONE',  ( 27.33329038210763784, 65.74999999999995737, -2.193932927905871022 ) ) ;
#2307=VERTEX_POINT ( 'NONE', #2583 ) ;
#2318=CARTESIAN_POINT ( 'NONE',  ( -28.41012295193859316, 51.34328577455362108, 1.513759717780124747 ) ) ;
#2319=AXIS2_PLACEMENT_3D ( 'NONE', #1178, #9418, #4561 ) ;
#2324=EDGE_LOOP ( 'NONE', ( #15752, #3083, #16575, #7086 ) ) ;
#2328=EDGE_LOOP ( 'NONE', ( #19910, #7756, #15014, #18546 ) ) ;
#2330=VERTEX_POINT ( 'NONE', #10823 ) ;
#2345=CARTESIAN_POINT ( 'NONE',  ( -33.44163564243958575, 75.56468634061936029, -1.801359935166299886 ) ) ;
#2356=DIRECTION ( 'NONE',  ( -0.8000000000000001554, 0.000000000000000000, -0.5999999999999999778 ) ) ;
#2360=CARTESIAN_POINT ( 'NONE',  ( -18.07408198074340788, 79.99963191228553683, -12.37854261456184268 ) ) ;
#2367=FACE_OUTER_BOUND ( 'NONE', #1220, .T. ) ;
#2374=ORIENTED_EDGE ( 'NONE', *, *, #11065, .T. ) ;
#2377=ORIENTED_EDGE ( 'NONE', *, *, #10708, .F. ) ;
#2378=EDGE_CURVE ( 'NONE', #20835, #4202, #7328, .T. ) ;
#2383=CARTESIAN_POINT ( 'NONE',  ( -28.41032686606757096, 6.478790711288843873, 1.559431153037987849 ) ) ;
#2390=CIRCLE ( 'NONE', #1034, 5.000000000000000888 ) ;
#2398=VERTEX_POINT ( 'NONE', #14355 ) ;
#2405=EDGE_LOOP ( 'NONE', ( #13727, #14907, #5786, #20302, #5911 ) ) ;
#2420=CARTESIAN_POINT ( 'NONE',  ( -25.43178678872172682, 45.02209116438434933, -8.210452674424425723 ) ) ;
#2427=CARTESIAN_POINT ( 'NONE',  ( -28.37382670920847971, 51.80430336678647762, 1.824942738421546862 ) ) ;
#2434=DIRECTION ( 'NONE',  ( 0.000000000000000000, -1.000000000000000000, 0.000000000000000000 ) ) ;
#2444=LINE ( 'NONE', #2758, #8385 ) ;
#2446=CARTESIAN_POINT ( 'NONE',  ( 30.10683012259193703, -10.00000000000000000, 0.000000000000000000 ) ) ;
#2453=CARTESIAN_POINT ( 'NONE',  ( -32.63107789565361117, 71.62317011047271365, 0.9609777548053090035 ) ) ;
#2459=CARTESIAN_POINT ( 'NONE',  ( -4.234137110339535326, 65.75000000000001421, 4.519411796990935315 ) ) ;
#2463=LINE ( 'NONE', #5512, #9142 ) ;
#2484=CARTESIAN_POINT ( 'NONE',  ( -4.701390418375630986, 65.75000000000000000, 5.347094680480811490 ) ) ;
#2496=CARTESIAN_POINT ( 'NONE',  ( -28.48629072751340630, 8.589818999910622921, -0.6763375131893898384 ) ) ;
#2501=AXIS2_PLACEMENT_3D ( 'NONE', #2446, #4136, #16855 ) ;
#2508=DIRECTION ( 'NONE',  ( -0.000000000000000000, -1.000000000000000000, 0.000000000000000000 ) ) ;
#2524=EDGE_CURVE ( 'NONE', #9666, #18381, #19939, .T. ) ;
#2528=CARTESIAN_POINT ( 'NONE',  ( -21.63303579789734243, 49.55866895486145296, -11.18335248048085084 ) ) ;
#2542=FACE_OUTER_BOUND ( 'NONE', #12900, .T. ) ;
#2543=CARTESIAN_POINT ( 'NONE',  ( 1.111705572786244156, 51.52592968046116084, -5.897422193562015913 ) ) ;
#2560=CARTESIAN_POINT ( 'NONE',  ( -28.86756580280676587, 70.94952981831229977, 1.317303739530243378 ) ) ;
#2565=CARTESIAN_POINT ( 'NONE',  ( -3.601011660222551036, 65.75000000000000000, 3.829121630900767848 ) ) ;
#2572=DIRECTION ( 'NONE',  ( 0.000000000000000000, 0.000000000000000000, -1.000000000000000000 ) ) ;
#2583=CARTESIAN_POINT ( 'NONE',  ( 26.99999999999999645, 65.74999999999995737, -2.528164662410434804 ) ) ;
#2601=CARTESIAN_POINT ( 'NONE',  ( -12.02901256816104336, 12.04372001624153476, 11.85403899944298622 ) ) ;
#2602=CARTESIAN_POINT ( 'NONE',  ( 10.49211908931699178, -10.00000000000000000, 5.000000000000000000 ) ) ;
#2607=CARTESIAN_POINT ( 'NONE',  ( 30.10683012259193703, 5.000000000000000000, 0.000000000000000000 ) ) ;
#2608=CARTESIAN_POINT ( 'NONE',  ( -15.99999999999999289, 80.00000000000000000, 0.000000000000000000 ) ) ;
#2624=CARTESIAN_POINT ( 'NONE',  ( -20.96748056867798837, 14.44039965061553410, 11.47079698816731685 ) ) ;
#2633=LINE ( 'NONE', #10772, #19364 ) ;
#2634=CARTESIAN_POINT ( 'NONE',  ( -15.66551832401957078, 45.63517971373708804, -12.50026680680302604 ) ) ;
#2638=CARTESIAN_POINT ( 'NONE',  ( -28.28813791240392916, 47.26616069107360829, -2.314127915140642866 ) ) ;
#2645=DIRECTION ( 'NONE',  ( 0.000000000000000000, 1.000000000000000000, 0.000000000000000000 ) ) ;
#2647=CARTESIAN_POINT ( 'NONE',  ( -15.23524979826371073, 50.47648804990845406, -16.25068009060050400 ) ) ;
#2648=CARTESIAN_POINT ( 'NONE',  ( -27.63586018514423515, 9.449117160379985947, -4.578843963689200436 ) ) ;
#2649=ORIENTED_EDGE ( 'NONE', *, *, #11330, .F. ) ;
#2659=CONICAL_SURFACE ( 'NONE', #14521, 9.999999999999998224, 0.7853981633974561616 ) ;
#2660=EDGE_CURVE ( 'NONE', #9451, #6871, #11535, .T. ) ;
#2665=CARTESIAN_POINT ( 'NONE',  ( 30.00000000000000355, 5.000000000000000000, -30.00000000000000000 ) ) ;
#2672=ORIENTED_EDGE ( 'NONE', *, *, #3004, .T. ) ;
#2675=EDGE_CURVE ( 'NONE', #4315, #5803, #710, .T. ) ;
#2679=EDGE_LOOP ( 'NONE', ( #12109, #14763, #15148, #3248, #16098, #14705, #10223, #8434, #14530, #18412 ) ) ;
#2682=FACE_BOUND ( 'NONE', #287, .T. ) ;
#2688=CARTESIAN_POINT ( 'NONE',  ( -12.45686459883834196, 60.55839683866341261, -3.534893197518178987 ) ) ;
#2691=CARTESIAN_POINT ( 'NONE',  ( -11.09026189855742572, 15.43276121221095920, 0.9457651797581775321 ) ) ;
#2702=DIRECTION ( 'NONE',  ( 1.000000000000000000, 0.000000000000000000, 0.000000000000000000 ) ) ;
#2708=ORIENTED_EDGE ( 'NONE', *, *, #13170, .T. ) ;
#2709=CARTESIAN_POINT ( 'NONE',  ( -34.00000000000000711, 65.74999999999997158, 2.481238266578629226 ) ) ;
#2711=CARTESIAN_POINT ( 'NONE',  ( 10.49211908931699178, 0.000000000000000000, 0.000000000000000000 ) ) ;
#2722=LINE ( 'NONE', #9162, #5113 ) ;
#2726=CARTESIAN_POINT ( 'NONE',  ( -17.30948708500259414, 10.26275758369035529, 12.43542173818663699 ) ) ;
#2734=CIRCLE ( 'NONE', #13920, 5.999999999999989342 ) ;
#2736=CARTESIAN_POINT ( 'NONE',  ( -18.73438247807179380, 45.53180543536074509, -12.20217720735596068 ) ) ;
#2739=CARTESIAN_POINT ( 'NONE',  ( -28.50078905930214290, 49.62758644748794978, 0.2159913647941864856 ) ) ;
#2741=ORIENTED_EDGE ( 'NONE', *, *, #13033, .F. ) ;
#2746=CARTESIAN_POINT ( 'NONE',  ( -2.766997014963338053, 76.74099499729231866, -3.129240771527075804 ) ) ;
#2752=CARTESIAN_POINT ( 'NONE',  ( -7.585160902965351504, 50.15125659263410540, -14.64997619612770485 ) ) ;
#2753=CARTESIAN_POINT ( 'NONE',  ( -26.41341864416630969, 9.999999999999992895, -6.948775141111584119 ) ) ;
#2756=CARTESIAN_POINT ( 'NONE',  ( 0.4195860999641303213, 70.63162242946638969, 1.437809060325977661 ) ) ;
#2758=CARTESIAN_POINT ( 'NONE',  ( 10.49211908931699178, 0.000000000000000000, 5.999999999999998224 ) ) ;
#2769=CARTESIAN_POINT ( 'NONE',  ( -31.85380967428733712, 66.50634452888658643, 2.432944671160833572 ) ) ;
#2778=CARTESIAN_POINT ( 'NONE',  ( -2.450339071221972365, 64.25000000000000000, 3.021668726329232779 ) ) ;
#2781=PRODUCT_CONTEXT ( 'NONE', #12849, 'mechanical' ) ;
#2784=DIRECTION ( 'NONE',  ( 0.000000000000000000, 0.000000000000000000, -1.000000000000000000 ) ) ;
#2786=DIRECTION ( 'NONE',  ( -0.000000000000000000, -1.000000000000000000, -0.000000000000000000 ) ) ;
#2796=FACE_OUTER_BOUND ( 'NONE', #12081, .T. ) ;
#2803=CARTESIAN_POINT ( 'NONE',  ( -33.32035108112687993, 77.22491497699215302, -3.799191488838269848 ) ) ;
#2807=EDGE_CURVE ( 'NONE', #4238, #13744, #12584, .T. ) ;
#2808=CARTESIAN_POINT ( 'NONE',  ( -11.00000000000000355, 15.09941697557068530, 11.45643923738960446 ) ) ;
#2813=CARTESIAN_POINT ( 'NONE',  ( -46.99999999999998579, 64.25000000000000000, -2.528164662410438357 ) ) ;
#2831=CARTESIAN_POINT ( 'NONE',  ( -17.62346795288569368, 10.35879774359155903, 12.39796379449725805 ) ) ;
#2841=CARTESIAN_POINT ( 'NONE',  ( -17.38132050553625518, 45.61375688610377921, -12.44240297365142567 ) ) ;
#2847=ORIENTED_EDGE ( 'NONE', *, *, #17548, .F. ) ;
#2848=EDGE_LOOP ( 'NONE', ( #9137, #10756, #20123 ) ) ;
#2850=DIRECTION ( 'NONE',  ( -0.000000000000000000, -0.000000000000000000, 1.000000000000000000 ) ) ;
#2856=CARTESIAN_POINT ( 'NONE',  ( 30.00000000000000355, 0.000000000000000000, -15.00000000000000000 ) ) ;
#2858=CARTESIAN_POINT ( 'NONE',  ( 0.9502985271742134810, 56.92418902563075278, 0.1464156901064357363 ) ) ;
#2859=DIRECTION ( 'NONE',  ( 0.000000000000000000, 0.000000000000000000, 1.000000000000000000 ) ) ;
#2869=CARTESIAN_POINT ( 'NONE',  ( -28.35076132082143374, 77.92717739396516663, 2.017250382391173158 ) ) ;
#2870=CARTESIAN_POINT ( 'NONE',  ( -20.74071588547708700, 16.72200274001069431, 11.56693563242971123 ) ) ;
#2873=DIRECTION ( 'NONE',  ( -0.000000000000000000, -1.000000000000000000, -0.000000000000000000 ) ) ;
#2875=AXIS2_PLACEMENT_3D ( 'NONE', #20016, #20118, #18639 ) ;
#2880=CARTESIAN_POINT ( 'NONE',  ( -3.050656336052146589, 73.64887869708235257, -0.2211343278613356611 ) ) ;
#2884=ORIENTED_EDGE ( 'NONE', *, *, #15899, .F. ) ;
#2891=LINE ( 'NONE', #17413, #15460 ) ;
#2899=CARTESIAN_POINT ( 'NONE',  ( -4.618023652948263447, 68.30950415664239017, 5.167706431871527784 ) ) ;
#2908=ADVANCED_FACE ( 'NONE', ( #11496 ), #13101, .T. ) ;
#2912=ADVANCED_FACE ( 'NONE', ( #3439 ), #11552, .F. ) ;
#2916=CARTESIAN_POINT ( 'NONE',  ( -15.99999999999999289, 15.09941697557068530, 0.9999999999999991118 ) ) ;
#2936=CIRCLE ( 'NONE', #20190, 4.999999999999997335 ) ;
#2943=CARTESIAN_POINT ( 'NONE',  ( -4.380992799470656784, 51.87686864743692894, -5.137587943657599077 ) ) ;
#2946=CARTESIAN_POINT ( 'NONE',  ( -27.35016751773910570, 45.66839489749002468, -5.250096803208007756 ) ) ;
#2958=CARTESIAN_POINT ( 'NONE',  ( -14.44414019777457092, 50.46616997920651215, -16.21138906647247779 ) ) ;
#2963=EDGE_CURVE ( 'NONE', #15695, #5066, #6124, .T. ) ;
#2992=DIRECTION ( 'NONE',  ( 0.000000000000000000, -1.000000000000000000, 0.000000000000000000 ) ) ;
#3004=EDGE_CURVE ( 'NONE', #10783, #3306, #3030, .T. ) ;
#3008=DIRECTION ( 'NONE',  ( 0.000000000000000000, -1.000000000000000000, 0.000000000000000000 ) ) ;
#3016=ADVANCED_FACE ( 'NONE', ( #5021, #3339 ), #16182, .T. ) ;
#3022=ADVANCED_FACE ( 'NONE', ( #1549 ), #20922, .T. ) ;
#3030=LINE ( 'NONE', #9474, #15975 ) ;
#3040=CARTESIAN_POINT ( 'NONE',  ( -4.715799786731095899, 45.61903957271908183, -5.387724600985420942 ) ) ;
#3049=CARTESIAN_POINT ( 'NONE',  ( -15.99999999999999289, 10.09941697557069418, 12.50000000000000000 ) ) ;
#3052=ORIENTED_EDGE ( 'NONE', *, *, #4691, .T. ) ;
#3057=CARTESIAN_POINT ( 'NONE',  ( -28.22616385396477057, 8.915032500921942216, 2.688307159736136764 ) ) ;
#3058=ORIENTED_EDGE ( 'NONE', *, *, #4826, .F. ) ;
#3068=AXIS2_PLACEMENT_3D ( 'NONE', #4984, #2140, #14673 ) ;
#3070=CARTESIAN_POINT ( 'NONE',  ( -31.81656357967666082, 64.12857799857799534, 2.491815815244385224 ) ) ;
#3073=VERTEX_POINT ( 'NONE', #19647 ) ;
#3083=ORIENTED_EDGE ( 'NONE', *, *, #5316, .T. ) ;
#3084=CARTESIAN_POINT ( 'NONE',  ( -3.117832412439754286, 75.18040026313899205, -1.430629151367028395 ) ) ;
#3094=ORIENTED_EDGE ( 'NONE', *, *, #3189, .F. ) ;
#3095=CARTESIAN_POINT ( 'NONE',  ( 30.10683012259193703, -24.14213562373095456, 0.000000000000000000 ) ) ;
#3101=DIRECTION ( 'NONE',  ( -0.000000000000000000, 1.000000000000000000, -0.000000000000000000 ) ) ;
#3116=CARTESIAN_POINT ( 'NONE',  ( -32.80236296842959121, 72.40585966223045489, 0.5537423545354294152 ) ) ;
#3119=CARTESIAN_POINT ( 'NONE',  ( -29.42634578414424240, 77.12664207850305331, -3.593879484355423592 ) ) ;
#3125=FACE_OUTER_BOUND ( 'NONE', #17314, .T. ) ;
#3130=ORIENTED_EDGE ( 'NONE', *, *, #3319, .T. ) ;
#3131=CIRCLE ( 'NONE', #17699, 12.50000000000000000 ) ;
#3141=CARTESIAN_POINT ( 'NONE',  ( -27.23257958228011688, 9.698350540763776451, -5.494722669932186498 ) ) ;
#3148=CARTESIAN_POINT ( 'NONE',  ( -3.660952356081173420, 47.48533333485243446, -2.023060265137478275 ) ) ;
#3156=CARTESIAN_POINT ( 'NONE',  ( -8.458929403065925001, 80.00000000014364332, -10.01181548797455889 ) ) ;
#3159=CARTESIAN_POINT ( 'NONE',  ( -19.01411426359141288, 59.74405275486697064, -3.991311237440302584 ) ) ;
#3161=CARTESIAN_POINT ( 'NONE',  ( -31.82323003959540486, 64.25000000000000000, 2.481238266578627449 ) ) ;
#3162=CARTESIAN_POINT ( 'NONE',  ( -11.81109483436797269, 62.83286948270322370, -2.731108915583023045 ) ) ;
#3171=LINE ( 'NONE', #14536, #15654 ) ;
#3176=CARTESIAN_POINT ( 'NONE',  ( -27.30495104032085862, 66.33121464498888997, 5.333703082177909671 ) ) ;
#3184=CARTESIAN_POINT ( 'NONE',  ( -4.120658645831395184, 73.83089348061646717, 3.891407385553233844 ) ) ;
#3189=EDGE_CURVE ( 'NONE', #11812, #4703, #8506, .T. ) ;
#3208=EDGE_CURVE ( 'NONE', #13235, #13711, #13595, .T. ) ;
#3210=ORIENTED_EDGE ( 'NONE', *, *, #20857, .T. ) ;
#3216=CARTESIAN_POINT ( 'NONE',  ( -25.79456020734900790, 80.00000000016163426, -7.778117258978351600 ) ) ;
#3229=ORIENTED_EDGE ( 'NONE', *, *, #4724, .F. ) ;
#3236=CARTESIAN_POINT ( 'NONE',  ( -30.00000000000023093, 4.999999999999890754, -7.265667520938737134 ) ) ;
#3242=CARTESIAN_POINT ( 'NONE',  ( -7.804814160866035522, 45.01037650073381968, -9.445069905521446429 ) ) ;
#3248=ORIENTED_EDGE ( 'NONE', *, *, #6523, .T. ) ;
#3252=CARTESIAN_POINT ( 'NONE',  ( -10.93912170749876722, 79.98244021547212412, -11.72107194671489339 ) ) ;
#3253=VERTEX_POINT ( 'NONE', #2602 ) ;
#3272=CARTESIAN_POINT ( 'NONE',  ( -32.65378408385129916, 58.26992351455638186, 0.9102417315387145713 ) ) ;
#3273=CARTESIAN_POINT ( 'NONE',  ( -20.99999999999998934, 15.26381062800292199, 11.45643923738960446 ) ) ;
#3281=VERTEX_POINT ( 'NONE', #12132 ) ;
#3287=VERTEX_POINT ( 'NONE', #8940 ) ;
#3293=MANIFOLD_SOLID_BREP ( 'Cut-Extrude9', #11357 ) ;
#3300=CARTESIAN_POINT ( 'NONE',  ( -15.99999999999999289, 0.000000000000000000, -5.999999999999989342 ) ) ;
#3301=EDGE_CURVE ( 'NONE', #8955, #13711, #8837, .T. ) ;
#3306=VERTEX_POINT ( 'NONE', #4800 ) ;
#3308=ADVANCED_FACE ( 'NONE', ( #16250 ), #6272, .F. ) ;
#3318=CARTESIAN_POINT ( 'NONE',  ( -33.99999999999997868, 64.25000000000000000, -2.528164662410438357 ) ) ;
#3319=EDGE_CURVE ( 'NONE', #11320, #9010, #4801, .T. ) ;
#3333=CARTESIAN_POINT ( 'NONE',  ( 30.00000000000000000, 0.000000000000000000, 28.99999999999999645 ) ) ;
#3336=EDGE_CURVE ( 'NONE', #17269, #3730, #3787, .T. ) ;
#3339=FACE_OUTER_BOUND ( 'NONE', #11473, .T. ) ;
#3341=CARTESIAN_POINT ( 'NONE',  ( -15.99999999999999289, 80.00000000000000000, 0.000000000000000000 ) ) ;
#3346=CARTESIAN_POINT ( 'NONE',  ( -4.095328035041411852, 55.94710214715788510, 3.823182773501264453 ) ) ;
#3348=VERTEX_POINT ( 'NONE', #19025 ) ;
#3349=CARTESIAN_POINT ( 'NONE',  ( -3.469238944213711040, 49.99908011708879485, -12.29405036578229549 ) ) ;
#3363=CARTESIAN_POINT ( 'NONE',  ( -15.11132063516011925, 58.47312285553441313, -4.923512665565291435 ) ) ;
#3380=CARTESIAN_POINT ( 'NONE',  ( -15.99999999999998934, 45.63508326896292289, -12.50000000000000000 ) ) ;
#3383=VERTEX_POINT ( 'NONE', #18823 ) ;
#3402=VERTEX_POINT ( 'NONE', #13740 ) ;
#3411=EDGE_LOOP ( 'NONE', ( #1971, #5989 ) ) ;
#3414=ORIENTED_EDGE ( 'NONE', *, *, #8756, .F. ) ;
#3416=EDGE_CURVE ( 'NONE', #10783, #3402, #2026, .T. ) ;
#3418=DIRECTION ( 'NONE',  ( 0.000000000000000000, -1.000000000000000000, 0.000000000000000000 ) ) ;
#3439=FACE_OUTER_BOUND ( 'NONE', #2007, .T. ) ;
#3450=CARTESIAN_POINT ( 'NONE',  ( -4.227323187870518417, 46.07367448256901099, -4.257085792854391038 ) ) ;
#3454=CARTESIAN_POINT ( 'NONE',  ( 1.463241080976594333, 52.61850491325280643, -4.024748401076783111 ) ) ;
#3457=EDGE_CURVE ( 'NONE', #3281, #17344, #18723, .T. ) ;
#3461=B_SPLINE_CURVE_WITH_KNOTS ( 'NONE', 3,
 ( #1970, #168, #13109, #2185, #3650, #19767, #19553, #19450, #18082, #8208, #18185, #16706, #8417, #10103, #16592, #8534, #15034, #17985, #3450, #493, #16393, #74, #6932, #18286, #13421, #1866, #5134, #8313, #19867, #3761, #10213, #3346, #17884, #1763, #9798, #269, #16287, #6714 ),
 .UNSPECIFIED., .F., .F.,
 ( 4, 2, 2, 2, 2, 2, 2, 2, 2, 2, 2, 2, 2, 2, 2, 2, 2, 2, 4 ),
 ( 0.03718627721641753342, 0.03834690901369668115, 0.03950754081097582887, 0.04182880440553412432, 0.04298943620281327205, 0.04415006800009241977, 0.04647133159465070829, 0.04879259518920900374, 0.05111385878376729919, 0.05343512237832559464, 0.05459575417560474236, 0.05575638597288389009, 0.05807764956744218554, 0.06039891316200048099, 0.06272017675655877644, 0.06504144035111705802, 0.06736270394567535347, 0.06968396754023364892, 0.07432649472935021207 ),
 .UNSPECIFIED. ) ;
#3481=EDGE_CURVE ( 'NONE', #13669, #11795, #8801, .T. ) ;
#3483=CARTESIAN_POINT ( 'NONE',  ( -28.43714190982515078, 50.99592196919532938, 1.276470960689417788 ) ) ;
#3488=CARTESIAN_POINT ( 'NONE',  ( -20.31374355284814825, 64.25000000000000000, -2.528164662410438357 ) ) ;
#3517=ORIENTED_EDGE ( 'NONE', *, *, #4758, .F. ) ;
#3534=DIRECTION ( 'NONE',  ( 0.6000000000000000888, 0.000000000000000000, 0.7999999999999999334 ) ) ;
#3548=ADVANCED_FACE ( 'NONE', ( #12469 ), #6078, .F. ) ;
#3553=CARTESIAN_POINT ( 'NONE',  ( -3.500383879130120501, 49.05626247071266732, -0.2969177088905650685 ) ) ;
#3563=VERTEX_POINT ( 'NONE', #18925 ) ;
#3569=CARTESIAN_POINT ( 'NONE',  ( -17.71827568934370234, 58.74352212083275759, -4.698501153746496684 ) ) ;
#3570=DIRECTION ( 'NONE',  ( -0.000000000000000000, 1.000000000000000000, -0.000000000000000000 ) ) ;
#3571=CARTESIAN_POINT ( 'NONE',  ( -12.00855099916729607, 61.81641395294881391, -3.013858250467857491 ) ) ;
#3577=ADVANCED_FACE ( 'NONE', ( #17443 ), #5977, .T. ) ;
#3578=VECTOR ( 'NONE', #7392, 1000.000000000000000 ) ;
#3579=AXIS2_PLACEMENT_3D ( 'NONE', #11778, #3920, #16653 ) ;
#3582=CARTESIAN_POINT ( 'NONE',  ( -33.28040837221767845, 51.87854031905991548, -5.222875071459978535 ) ) ;
#3583=CARTESIAN_POINT ( 'NONE',  ( -18.22437098228045116, 19.58037170849552311, 12.30137062747990306 ) ) ;
#3599=CARTESIAN_POINT ( 'NONE',  ( -4.701390418375630986, 65.75000000000000000, 5.347094680480811490 ) ) ;
#3614=CARTESIAN_POINT ( 'NONE',  ( 30.00000000000000355, -10.00000000000000000, -30.00000000000000000 ) ) ;
#3617=ORIENTED_EDGE ( 'NONE', *, *, #3481, .T. ) ;
#3624=CARTESIAN_POINT ( 'NONE',  ( -24.58391324610231266, 79.99999999992814992, -9.098350519373951784 ) ) ;
#3626=DIRECTION ( 'NONE',  ( -0.000000000000000000, 1.000000000000000000, -0.000000000000000000 ) ) ;
#3637=DIRECTION ( 'NONE',  ( 0.000000000000000000, 0.000000000000000000, 1.000000000000000000 ) ) ;
#3638=CARTESIAN_POINT ( 'NONE',  ( -6.118771807841490329, 79.85840876778712527, -10.43301765575355233 ) ) ;
#3641=FACE_OUTER_BOUND ( 'NONE', #11418, .T. ) ;
#3650=CARTESIAN_POINT ( 'NONE',  ( -14.06953418112486887, 45.58387777135212815, -12.35599831547759742 ) ) ;
#3654=CARTESIAN_POINT ( 'NONE',  ( 1.431553936783702685, 52.41835994622631745, -4.324939117741945616 ) ) ;
#3655=CARTESIAN_POINT ( 'NONE',  ( -6.896700228544379030, 79.90031512599163932, -10.76368999076717436 ) ) ;
#3676=ADVANCED_FACE ( 'NONE', ( #18269 ), #8402, .F. ) ;
#3678=CARTESIAN_POINT ( 'NONE',  ( -27.92487288654064059, 52.24757969830196203, -4.564036982978468160 ) ) ;
#3682=DIRECTION ( 'NONE',  ( -0.000000000000000000, -1.000000000000000000, -0.000000000000000000 ) ) ;
#3688=EDGE_CURVE ( 'NONE', #4749, #8514, #18609, .T. ) ;
#3712=CARTESIAN_POINT ( 'NONE',  ( -1.794545525815418596, 65.74999999999998579, 2.744335235139482965 ) ) ;
#3715=CARTESIAN_POINT ( 'NONE',  ( -12.09671107471471707, 68.50841174652784105, -3.129485610713131027 ) ) ;
#3720=AXIS2_PLACEMENT_3D ( 'NONE', #14151, #14365, #11055 ) ;
#3721=ORIENTED_EDGE ( 'NONE', *, *, #9073, .F. ) ;
#3726=CARTESIAN_POINT ( 'NONE',  ( -16.26048471067390011, 79.99999999999998579, -12.50000000001717204 ) ) ;
#3730=VERTEX_POINT ( 'NONE', #18068 ) ;
#3732=VECTOR ( 'NONE', #19608, 1000.000000000000000 ) ;
#3737=DIRECTION ( 'NONE',  ( 0.000000000000000000, 0.000000000000000000, 1.000000000000000000 ) ) ;
#3740=CYLINDRICAL_SURFACE ( 'NONE', #13952, 4.999999999999997335 ) ;
#3741=CARTESIAN_POINT ( 'NONE',  ( -5.443139766541319702, 79.99999999967708675, -6.747797645777612097 ) ) ;
#3744=ORIENTED_EDGE ( 'NONE', *, *, #9979, .T. ) ;
#3745=DIRECTION ( 'NONE',  ( 0.000000000000000000, 0.000000000000000000, 1.000000000000000000 ) ) ;
#3752=CARTESIAN_POINT ( 'NONE',  ( -29.99999999999999645, 5.000000000000000000, 6.407083732717120839 ) ) ;
#3761=CARTESIAN_POINT ( 'NONE',  ( -3.843826630376830256, 53.82522964764072526, 2.934722157913033591 ) ) ;
#3764=CARTESIAN_POINT ( 'NONE',  ( 0.08412497154685684431, 61.29016009911742202, 2.051811571683283653 ) ) ;
#3765=CARTESIAN_POINT ( 'NONE',  ( -4.367998177332779619, 79.71679007096339831, -9.567661261929613303 ) ) ;
#3770=LINE ( 'NONE', #278, #19793 ) ;
#3784=CARTESIAN_POINT ( 'NONE',  ( -15.99999999999999289, 65.74999999999998579, 0.000000000000000000 ) ) ;
#3787=CIRCLE ( 'NONE', #9196, 13.99999999999999822 ) ;
#3791=CARTESIAN_POINT ( 'NONE',  ( -26.37630993324036766, 50.77084747640196127, -7.029141103310240446 ) ) ;
#3792=CARTESIAN_POINT ( 'NONE',  ( -18.07496646850146149, 19.65148331647667845, 12.32752590463885412 ) ) ;
#3807=CARTESIAN_POINT ( 'NONE',  ( -15.99999999999999289, 9.999999999999994671, 0.000000000000000000 ) ) ;
#3808=B_SPLINE_CURVE_WITH_KNOTS ( 'NONE', 3,
 ( #16729, #5676, #18736, #10447, #8868, #12165, #3999, #10560, #20003, #615, #17045, #2206, #19893, #18629, #8663, #8766, #11962, #4210, #13866, #10654 ),
 .UNSPECIFIED., .F., .F.,
 ( 4, 2, 2, 2, 2, 2, 2, 2, 2, 4 ),
 ( 0.008555345346386189487, 0.009089294358497951309, 0.009623243370609713132, 0.01069114139483322810, 0.01175903941905674134, 0.01282693744328025631, 0.01389483546750376781, 0.01496273349172728279, 0.01603063151595079602, 0.01709852954017430926 ),
 .UNSPECIFIED. ) ;
#3815=CARTESIAN_POINT ( 'NONE',  ( -35.00000000000000000, 65.00000000000000000, -12.50000000000000000 ) ) ;
#3818=AXIS2_PLACEMENT_3D ( 'NONE', #4217, #17051, #17151 ) ;
#3825=CARTESIAN_POINT ( 'NONE',  ( -4.701390418375630986, 65.75000000000000000, 5.347094680480811490 ) ) ;
#3836=CARTESIAN_POINT ( 'NONE',  ( -25.88122819216030024, 79.85840876778742370, -10.43301765575532514 ) ) ;
#3837=LINE ( 'NONE', #7012, #17778 ) ;
#3839=EDGE_CURVE ( 'NONE', #13750, #12912, #15329, .T. ) ;
#3840=ORIENTED_EDGE ( 'NONE', *, *, #1283, .T. ) ;
#3846=ORIENTED_EDGE ( 'NONE', *, *, #15147, .T. ) ;
#3857=CARTESIAN_POINT ( 'NONE',  ( 10.49211908931699178, -10.00000000000000000, 0.000000000000000000 ) ) ;
#3862=CARTESIAN_POINT ( 'NONE',  ( -25.99999999999999289, 4.999999999999994671, 7.500000000000009770 ) ) ;
#3871=CARTESIAN_POINT ( 'NONE',  ( 28.00000000000001066, 64.25000000000000000, 75.00000000000000000 ) ) ;
#3895=CARTESIAN_POINT ( 'NONE',  ( -26.75428091535899000, 51.05733496925417825, -6.497914592029476744 ) ) ;
#3910=CIRCLE ( 'NONE', #9655, 13.99999999999999822 ) ;
#3917=CARTESIAN_POINT ( 'NONE',  ( 0.000000000000000000, -10.00000000000000000, 0.000000000000000000 ) ) ;
#3920=DIRECTION ( 'NONE',  ( 0.000000000000000000, -1.000000000000000000, 0.000000000000000000 ) ) ;
#3944=CARTESIAN_POINT ( 'NONE',  ( -24.90922013266621704, 80.00000000007942447, -8.779353540718402016 ) ) ;
#3947=ADVANCED_FACE ( 'NONE', ( #15741 ), #12656, .F. ) ;
#3949=DIRECTION ( 'NONE',  ( 0.000000000000000000, 0.000000000000000000, -1.000000000000000000 ) ) ;
#3951=SHAPE_REPRESENTATION ( 'Base Lock Knob', ( #18233 ), #6025 ) ;
#3953=DIRECTION ( 'NONE',  ( 6.608470384673549052E-16, -1.000000000000000000, 0.000000000000000000 ) ) ;
#3967=CARTESIAN_POINT ( 'NONE',  ( -15.99999999999999289, 9.999999999999994671, 0.000000000000000000 ) ) ;
#3969=CARTESIAN_POINT ( 'NONE',  ( -30.00000000000019895, 4.999999999999801048, -0.4747169640371201038 ) ) ;
#3974=CIRCLE ( 'NONE', #11089, 15.00000000000000000 ) ;
#3977=VECTOR ( 'NONE', #12881, 1000.000000000000000 ) ;
#3980=DIRECTION ( 'NONE',  ( 0.000000000000000000, 0.000000000000000000, 1.000000000000000000 ) ) ;
#3999=CARTESIAN_POINT ( 'NONE',  ( -17.72229213209295651, 71.26752244718856844, -4.704935945893314653 ) ) ;
#4003=CARTESIAN_POINT ( 'NONE',  ( -29.51915980583113353, 50.03287237322234660, -11.46702022756807970 ) ) ;
#4006=CARTESIAN_POINT ( 'NONE',  ( -28.07387375345178882, 54.51268698003941893, 3.249670041809122889 ) ) ;
#4007=ORIENTED_EDGE ( 'NONE', *, *, #9229, .T. ) ;
#4008=ORIENTED_EDGE ( 'NONE', *, *, #12277, .F. ) ;
#4017=ORIENTED_EDGE ( 'NONE', *, *, #14339, .F. ) ;
#4023=CARTESIAN_POINT ( 'NONE',  ( -12.94355555882016162, 19.06978034970748226, 12.12372807873016711 ) ) ;
#4054=ORIENTED_EDGE ( 'NONE', *, *, #3688, .T. ) ;
#4068=CARTESIAN_POINT ( 'NONE',  ( -33.07648103134474837, 77.63984378200004244, -4.412136689679511115 ) ) ;
#4071=CARTESIAN_POINT ( 'NONE',  ( -29.99999999999999645, -10.00000000000000000, -15.00000000000000000 ) ) ;
#4072=CARTESIAN_POINT ( 'NONE',  ( -28.48162945689469083, 6.472597147970983400, -0.7888061438404905257 ) ) ;
#4087=CARTESIAN_POINT ( 'NONE',  ( -34.66668267600675080, 64.25000000000000000, 1.813692929321156333 ) ) ;
#4088=DIRECTION ( 'NONE',  ( -0.000000000000000000, 1.000000000000000000, -0.000000000000000000 ) ) ;
#4094=ADVANCED_FACE ( 'NONE', ( #4896, #9659 ), #336, .T. ) ;
#4102=ADVANCED_FACE ( 'NONE', ( #4988 ), #1823, .F. ) ;
#4104=FACE_BOUND ( 'NONE', #18020, .T. ) ;
#4112=CARTESIAN_POINT ( 'NONE',  ( -23.47727273277572380, 50.20802583047444756, -15.01355377214448517 ) ) ;
#4114=VECTOR ( 'NONE', #580, 1000.000000000000000 ) ;
#4117=CARTESIAN_POINT ( 'NONE',  ( -27.66274264245146242, 58.14439702606364335, 4.503690111865336299 ) ) ;
#4124=VERTEX_POINT ( 'NONE', #14780 ) ;
#4127=CARTESIAN_POINT ( 'NONE',  ( 0.4725499000616883993, 50.80107947907877985, -7.614411031363864879 ) ) ;
#4136=DIRECTION ( 'NONE',  ( -0.000000000000000000, 1.000000000000000000, -0.000000000000000000 ) ) ;
#4137=CARTESIAN_POINT ( 'NONE',  ( -15.34316709825168168, 20.06719728497707678, 12.48700296046530411 ) ) ;
#4140=CARTESIAN_POINT ( 'NONE',  ( -27.95542020482363199, 74.48392764733534932, 3.658293529343086270 ) ) ;
#4141=CARTESIAN_POINT ( 'NONE',  ( -20.99999999999998934, 15.09941697557068530, 0.9999999999999991118 ) ) ;
#4142=EDGE_LOOP ( 'NONE', ( #14421, #653, #5770, #12835 ) ) ;
#4143=CARTESIAN_POINT ( 'NONE',  ( -32.77872921741722223, 72.29984585682672105, 0.6063817381316165545 ) ) ;
#4144=CARTESIAN_POINT ( 'NONE',  ( -20.31374355284814825, 65.74999999999995737, -2.528164662410434804 ) ) ;
#4162=PLANE ( 'NONE',  #1199 ) ;
#4171=CARTESIAN_POINT ( 'NONE',  ( -4.044579795176349357, 74.48392764733533511, 3.658293529343076500 ) ) ;
#4172=EDGE_CURVE ( 'NONE', #16360, #1288, #7532, .T. ) ;
#4192=CARTESIAN_POINT ( 'NONE',  ( 30.10683012259193703, -10.00000000000000000, -4.999999999999997335 ) ) ;
#4196=DIRECTION ( 'NONE',  ( -0.000000000000000000, -0.000000000000000000, 1.000000000000000000 ) ) ;
#4202=VERTEX_POINT ( 'NONE', #4225 ) ;
#4210=CARTESIAN_POINT ( 'NONE',  ( -20.27070155495306025, 66.46434188593948988, -2.601344003386939718 ) ) ;
#4213=CARTESIAN_POINT ( 'NONE',  ( 26.99999999999999645, 65.00000000000000000, -22.50000000000000000 ) ) ;
#4216=CARTESIAN_POINT ( 'NONE',  ( -21.00073344079603999, 49.53628891258126998, -11.48274257968635759 ) ) ;
#4217=CARTESIAN_POINT ( 'NONE',  ( -33.99999999999997868, 65.00000000000000000, -12.50000000000000000 ) ) ;
#4222=VERTEX_POINT ( 'NONE', #1258 ) ;
#4225=CARTESIAN_POINT ( 'NONE',  ( -11.09026189855725164, 15.09941697557061957, 0.9457651797582804498 ) ) ;
#4226=CARTESIAN_POINT ( 'NONE',  ( 1.484819526751606000, 76.25000000000000000, -2.578432583507790810 ) ) ;
#4232=CARTESIAN_POINT ( 'NONE',  ( 1.204199731550535946, 51.70050625791687082, -5.552164477314467383 ) ) ;
#4233=PLANE ( 'NONE',  #18156 ) ;
#4238=VERTEX_POINT ( 'NONE', #11105 ) ;
#4245=DIRECTION ( 'NONE',  ( -0.000000000000000000, -0.000000000000000000, 1.000000000000000000 ) ) ;
#4248=CARTESIAN_POINT ( 'NONE',  ( -28.62307079896444506, 76.35052269458219598, -2.692414605357470681 ) ) ;
#4266=CARTESIAN_POINT ( 'NONE',  ( -15.99999999999999289, 80.00000000000000000, -12.50000000000000000 ) ) ;
#4279=DIRECTION ( 'NONE',  ( 0.000000000000000000, 0.000000000000000000, -1.000000000000000000 ) ) ;
#4290=CARTESIAN_POINT ( 'NONE',  ( -35.00000000000000000, 64.25000000000000000, 2.481238266578627449 ) ) ;
#4298=CARTESIAN_POINT ( 'NONE',  ( 28.00000000000001066, 65.75000000000001421, -1.525597966175989972 ) ) ;
#4300=DIRECTION ( 'NONE',  ( -0.000000000000000000, 1.000000000000000000, -0.000000000000000000 ) ) ;
#4307=ORIENTED_EDGE ( 'NONE', *, *, #8901, .F. ) ;
#4315=VERTEX_POINT ( 'NONE', #15483 ) ;
#4316=AXIS2_PLACEMENT_3D ( 'NONE', #14588, #9575, #9677 ) ;
#4320=CARTESIAN_POINT ( 'NONE',  ( -19.82813546932964144, 50.39885407664990424, -15.93728606778036649 ) ) ;
#4334=DIRECTION ( 'NONE',  ( 0.000000000000000000, 0.000000000000000000, 1.000000000000000000 ) ) ;
#4336=CARTESIAN_POINT ( 'NONE',  ( 0.6561171340770418636, 58.25694778279074626, 0.9210584346784731480 ) ) ;
#4337=CARTESIAN_POINT ( 'NONE',  ( -27.23510498666222546, 9.696991385916662765, -5.489464333053563294 ) ) ;
#4341=CARTESIAN_POINT ( 'NONE',  ( 0.8023629684295970899, 72.40585966223045489, 0.5537423545354359655 ) ) ;
#4360=CARTESIAN_POINT ( 'NONE',  ( -3.055511853597258742, 64.25000000000000000, 3.385962996190660768 ) ) ;
#4369=DIRECTION ( 'NONE',  ( 0.000000000000000000, -0.000000000000000000, -1.000000000000000000 ) ) ;
#4384=CARTESIAN_POINT ( 'NONE',  ( -33.46953329182479564, 76.75544209468823453, -3.174647668799659872 ) ) ;
#4385=ADVANCED_FACE ( 'NONE', ( #90 ), #6729, .T. ) ;
#4389=DIRECTION ( 'NONE',  ( 0.000000000000000000, 0.000000000000000000, -1.000000000000000000 ) ) ;
#4418=DIRECTION ( 'NONE',  ( 1.000000000000000000, -0.000000000000000000, -0.000000000000000000 ) ) ;
#4422=CARTESIAN_POINT ( 'NONE',  ( -19.99008258158868756, 49.51761908642668431, -11.85432026588631338 ) ) ;
#4425=CARTESIAN_POINT ( 'NONE',  ( -28.44688792319594128, 50.84930382153548578, 1.171743096592904765 ) ) ;
#4436=ORIENTED_EDGE ( 'NONE', *, *, #4972, .F. ) ;
#4437=EDGE_CURVE ( 'NONE', #2398, #1492, #8827, .T. ) ;
#4440=CARTESIAN_POINT ( 'NONE',  ( -3.198494086879704934, 50.00375224366489846, -12.08029061943339322 ) ) ;
#4441=CARTESIAN_POINT ( 'NONE',  ( -25.99999999999999645, 9.999999999999994671, 7.500000000000000000 ) ) ;
#4444=ADVANCED_FACE ( 'NONE', ( #285 ), #6522, .T. ) ;
#4446=CARTESIAN_POINT ( 'NONE',  ( 1.317725315667332309, 74.84505238333373711, -1.139833306050669126 ) ) ;
#4448=AXIS2_PLACEMENT_3D ( 'NONE', #20388, #18915, #4389 ) ;
#4455=DIRECTION ( 'NONE',  ( 0.000000000000000000, 0.000000000000000000, -1.000000000000000000 ) ) ;
#4470=CARTESIAN_POINT ( 'NONE',  ( 0.7787292174182174342, 72.29984585682862530, 0.6063817381306070287 ) ) ;
#4478=DIRECTION ( 'NONE',  ( 1.000000000000000000, 0.000000000000000000, 0.000000000000000000 ) ) ;
#4479=CARTESIAN_POINT ( 'NONE',  ( -11.10102051443364779, 14.09941697557065332, 0.9999999999999991118 ) ) ;
#4492=DIRECTION ( 'NONE',  ( -0.000000000000000000, -0.000000000000000000, 1.000000000000000000 ) ) ;
#4497=CARTESIAN_POINT ( 'NONE',  ( -14.69480916118295255, 10.26995882791192471, 12.43268610818004838 ) ) ;
#4501=ADVANCED_FACE ( 'NONE', ( #10439 ), #2075, .F. ) ;
#4509=ORIENTED_EDGE ( 'NONE', *, *, #11330, .T. ) ;
#4514=CARTESIAN_POINT ( 'NONE',  ( -15.99999999999999289, 9.999999999999994671, 0.000000000000000000 ) ) ;
#4530=CARTESIAN_POINT ( 'NONE',  ( -4.094320337108634966, 46.27675487045426905, -3.861523532182237428 ) ) ;
#4533=CARTESIAN_POINT ( 'NONE',  ( -24.14678699472350587, 45.01203632813575695, -9.488349599000542867 ) ) ;
#4536=ORIENTED_EDGE ( 'NONE', *, *, #12483, .F. ) ;
#4544=CARTESIAN_POINT ( 'NONE',  ( -4.472320007499605232, 50.00706524506586703, -13.00541661879220356 ) ) ;
#4545=CARTESIAN_POINT ( 'NONE',  ( -28.43148821208374244, 8.662657545001765769, 1.350916757379553967 ) ) ;
#4548=CARTESIAN_POINT ( 'NONE',  ( 0.02492996559929827605, 68.25592811474754740, 2.150873336511314626 ) ) ;
#4550=( NAMED_UNIT ( * ) PLANE_ANGLE_UNIT ( ) SI_UNIT ( $, .RADIAN. ) );
#4560=ORIENTED_EDGE ( 'NONE', *, *, #15377, .T. ) ;
#4561=DIRECTION ( 'NONE',  ( 0.000000000000000000, 0.000000000000000000, -1.000000000000000000 ) ) ;
#4563=FACE_OUTER_BOUND ( 'NONE', #13048, .T. ) ;
#4564=VERTEX_POINT ( 'NONE', #8860 ) ;
#4568=CARTESIAN_POINT ( 'NONE',  ( -3.979955202765648181, 75.03053098945672161, 3.432994178268343965 ) ) ;
#4570=DIRECTION ( 'NONE',  ( 0.000000000000000000, -1.000000000000000000, 0.000000000000000000 ) ) ;
#4579=DIRECTION ( 'NONE',  ( -0.000000000000000000, 1.000000000000000000, -0.000000000000000000 ) ) ;
#4594=DIRECTION ( 'NONE',  ( 0.000000000000000000, 0.000000000000000000, -1.000000000000000000 ) ) ;
#4596=VERTEX_POINT ( 'NONE', #6949 ) ;
#4611=DIRECTION ( 'NONE',  ( -0.000000000000000000, -1.000000000000000000, -0.000000000000000000 ) ) ;
#4630=CARTESIAN_POINT ( 'NONE',  ( -7.082764429467357736, 50.04906111657209067, -8.763765402883818112 ) ) ;
#4637=ORIENTED_EDGE ( 'NONE', *, *, #5054, .F. ) ;
#4639=FACE_OUTER_BOUND ( 'NONE', #14377, .T. ) ;
#4647=DIRECTION ( 'NONE',  ( -0.000000000000000000, 1.000000000000000000, -0.000000000000000000 ) ) ;
#4648=CARTESIAN_POINT ( 'NONE',  ( -32.10259343984367320, 61.14548605613433097, 2.017374915500129706 ) ) ;
#4649=CARTESIAN_POINT ( 'NONE',  ( -28.48674344962430283, 8.589208059839100073, 0.6694126349350221217 ) ) ;
#4651=ORIENTED_EDGE ( 'NONE', *, *, #1914, .T. ) ;
#4656=CARTESIAN_POINT ( 'NONE',  ( -27.42628672828266545, 60.97609658108721931, 5.069224955254768794 ) ) ;
#4665=EDGE_LOOP ( 'NONE', ( #17748, #9634, #16786, #4008 ) ) ;
#4666=CARTESIAN_POINT ( 'NONE',  ( -3.297392717249913119, 67.76582539289996987, 2.255487788202362509 ) ) ;
#4685=VECTOR ( 'NONE', #16040, 1000.000000000000000 ) ;
#4687=VERTEX_POINT ( 'NONE', #9663 ) ;
#4691=EDGE_CURVE ( 'NONE', #17545, #4687, #14368, .T. ) ;
#4692=ORIENTED_EDGE ( 'NONE', *, *, #8214, .T. ) ;
#4698=ORIENTED_EDGE ( 'NONE', *, *, #10799, .F. ) ;
#4700=CARTESIAN_POINT ( 'NONE',  ( -28.42369844106826093, 79.61691370731600159, -9.098688494702861007 ) ) ;
#4703=VERTEX_POINT ( 'NONE', #15945 ) ;
#4713=ORIENTED_EDGE ( 'NONE', *, *, #13910, .T. ) ;
#4719=DIRECTION ( 'NONE',  ( 0.000000000000000000, -0.000000000000000000, -1.000000000000000000 ) ) ;
#4722=CARTESIAN_POINT ( 'NONE',  ( -29.99999999999999645, 5.000000000000000000, -15.00000000000000000 ) ) ;
#4724=EDGE_CURVE ( 'NONE', #12607, #245, #916, .T. ) ;
#4729=CARTESIAN_POINT ( 'NONE',  ( -10.39101401679802450, 49.56263860070575333, -11.18078835284466344 ) ) ;
#4734=DIRECTION ( 'NONE',  ( -1.000000000000000000, 0.000000000000000000, 0.000000000000000000 ) ) ;
#4737=CARTESIAN_POINT ( 'NONE',  ( 28.00000000000001066, 65.00000000000000000, -23.50000000000002842 ) ) ;
#4740=CARTESIAN_POINT ( 'NONE',  ( -14.69985738491135052, 80.00000000000054001, -12.43489149392604887 ) ) ;
#4741=EDGE_LOOP ( 'NONE', ( #7977, #18174 ) ) ;
#4749=VERTEX_POINT ( 'NONE', #17035 ) ;
#4750=CARTESIAN_POINT ( 'NONE',  ( 30.00000000000000355, -9.999999999999998224, -15.00000000000000000 ) ) ;
#4755=CARTESIAN_POINT ( 'NONE',  ( -28.64932889238898284, 64.82996465168147893, 2.499044199174691450 ) ) ;
#4758=EDGE_CURVE ( 'NONE', #17545, #20090, #19221, .T. ) ;
#4759=CARTESIAN_POINT ( 'NONE',  ( -28.66754328919736849, 66.65723886915071716, 2.419320319690952292 ) ) ;
#4762=CARTESIAN_POINT ( 'NONE',  ( 10.49211908931699178, 0.000000000000000000, -5.999999999999998224 ) ) ;
#4768=CARTESIAN_POINT ( 'NONE',  ( 1.064779251448269903, 73.59974835484908340, -0.1995438761926260351 ) ) ;
#4779=CYLINDRICAL_SURFACE ( 'NONE', #6020, 4.999999999999997335 ) ;
#4789=CARTESIAN_POINT ( 'NONE',  ( 30.00000000000000355, 0.000000000000000000, -28.99999999999999645 ) ) ;
#4790=ORIENTED_EDGE ( 'NONE', *, *, #12277, .T. ) ;
#4793=DIRECTION ( 'NONE',  ( 1.000000000000000000, 0.000000000000000000, 0.000000000000000000 ) ) ;
#4794=AXIS2_PLACEMENT_3D ( 'NONE', #8620, #8725, #7024 ) ;
#4796=DIRECTION ( 'NONE',  ( 0.000000000000000000, -1.000000000000000000, 0.000000000000000000 ) ) ;
#4800=CARTESIAN_POINT ( 'NONE',  ( -35.00000000000000000, 64.25000000000000000, -1.525597966176003961 ) ) ;
#4801=CIRCLE ( 'NONE', #75, 11.00000000000002665 ) ;
#4806=CARTESIAN_POINT ( 'NONE',  ( -30.24532165557386421, 79.23832348577512619, -7.772177369788165535 ) ) ;
#4826=EDGE_CURVE ( 'NONE', #11812, #9209, #15886, .T. ) ;
#4833=ORIENTED_EDGE ( 'NONE', *, *, #7680, .T. ) ;
#4835=CARTESIAN_POINT ( 'NONE',  ( -4.309763885322762889, 45.97587668858208332, -4.475643294533367289 ) ) ;
#4839=CARTESIAN_POINT ( 'NONE',  ( -24.99005427693084158, 44.99862682014547488, -8.693708486900669996 ) ) ;
#4844=CARTESIAN_POINT ( 'NONE',  ( -13.92591801928538686, 79.99963191531476525, -12.37854261419849422 ) ) ;
#4852=CARTESIAN_POINT ( 'NONE',  ( -11.70208324916672815, 63.89094914002017589, -2.555169535221542887 ) ) ;
#4863=CARTESIAN_POINT ( 'NONE',  ( -32.09082692128702519, 61.27974766235208648, 2.035803694763616445 ) ) ;
#4864=CARTESIAN_POINT ( 'NONE',  ( 45.00000000000000000, 5.000000000000000000, -15.00000000000000000 ) ) ;
#4880=VERTEX_POINT ( 'NONE', #3614 ) ;
#4896=FACE_BOUND ( 'NONE', #12073, .T. ) ;
#4902=DIRECTION ( 'NONE',  ( 0.000000000000000000, 0.000000000000000000, -1.000000000000000000 ) ) ;
#4912=VERTEX_POINT ( 'NONE', #1935 ) ;
#4925=CARTESIAN_POINT ( 'NONE',  ( -28.38973003226371006, 8.717107242880045348, -1.690292246971881740 ) ) ;
#4934=CARTESIAN_POINT ( 'NONE',  ( -6.351643513575302435, 45.03196607589810441, -7.976803885185221432 ) ) ;
#4935=CARTESIAN_POINT ( 'NONE',  ( -0.4023781907215778220, 78.75502016293279439, -6.506953707587063818 ) ) ;
#4938=CARTESIAN_POINT ( 'NONE',  ( -23.23502873769109556, 45.07676717092099494, -10.20065155966471337 ) ) ;
#4947=CARTESIAN_POINT ( 'NONE',  ( -18.57020691453844208, 59.27322340592550631, -4.297493274131830354 ) ) ;
#4954=ORIENTED_EDGE ( 'NONE', *, *, #3336, .F. ) ;
#4955=AXIS2_PLACEMENT_3D ( 'NONE', #14187, #19050, #17453 ) ;
#4963=CARTESIAN_POINT ( 'NONE',  ( 27.00000000000002487, 65.74999999999997158, 2.481238266578629226 ) ) ;
#4966=ORIENTED_EDGE ( 'NONE', *, *, #358, .T. ) ;
#4972=EDGE_CURVE ( 'NONE', #19075, #6984, #13700, .T. ) ;
#4979=DIRECTION ( 'NONE',  ( 0.000000000000000000, -1.000000000000000000, 0.000000000000000000 ) ) ;
#4984=CARTESIAN_POINT ( 'NONE',  ( 28.00000000000001066, 65.00000000000000000, -12.50000000000000000 ) ) ;
#4988=FACE_OUTER_BOUND ( 'NONE', #13675, .T. ) ;
#5002=CARTESIAN_POINT ( 'NONE',  ( -27.98085110631299344, 80.00000000015971580, -3.582299587997329837 ) ) ;
#5004=EDGE_CURVE ( 'NONE', #6727, #8661, #2463, .T. ) ;
#5012=ORIENTED_EDGE ( 'NONE', *, *, #7026, .F. ) ;
#5017=CARTESIAN_POINT ( 'NONE',  ( -14.99999999999999645, 5.000000000000000000, 15.00000000000000000 ) ) ;
#5021=FACE_BOUND ( 'NONE', #3411, .T. ) ;
#5034=CARTESIAN_POINT ( 'NONE',  ( -3.616241391857264009, 47.72147621156500463, -1.725877097790484704 ) ) ;
#5043=DIRECTION ( 'NONE',  ( 1.000000000000000000, 0.000000000000000000, 0.000000000000000000 ) ) ;
#5054=EDGE_CURVE ( 'NONE', #15623, #9666, #12844, .T. ) ;
#5059=CARTESIAN_POINT ( 'NONE',  ( -32.38649895722338812, 50.74460817506653143, -7.785217389867390203 ) ) ;
#5066=VERTEX_POINT ( 'NONE', #1292 ) ;
#5099=AXIS2_PLACEMENT_3D ( 'NONE', #1983, #9910, #8431 ) ;
#5100=ADVANCED_FACE ( 'NONE', ( #20870 ), #13688, .F. ) ;
#5104=ORIENTED_EDGE ( 'NONE', *, *, #5853, .F. ) ;
#5105=CARTESIAN_POINT ( 'NONE',  ( 10.49211908931699178, 0.000000000000000000, -5.999999999999998224 ) ) ;
#5111=AXIS2_PLACEMENT_3D ( 'NONE', #9397, #2645, #20538 ) ;
#5113=VECTOR ( 'NONE', #7472, 1000.000000000000000 ) ;
#5116=ORIENTED_EDGE ( 'NONE', *, *, #13957, .F. ) ;
#5119=CARTESIAN_POINT ( 'NONE',  ( 30.00000000000000000, 5.000000000000000000, 15.00000000000000000 ) ) ;
#5129=CARTESIAN_POINT ( 'NONE',  ( -27.41869751006752409, 6.332780952808748864, -5.130582469439492144 ) ) ;
#5134=CARTESIAN_POINT ( 'NONE',  ( -3.528418202498509348, 50.52477872402794645, 0.9493153023570927163 ) ) ;
#5137=CARTESIAN_POINT ( 'NONE',  ( -3.989626255526430132, 52.36474351664826798, -4.388076984466315444 ) ) ;
#5140=VECTOR ( 'NONE', #1303, 1000.000000000000000 ) ;
#5147=ORIENTED_EDGE ( 'NONE', *, *, #14759, .F. ) ;
#5152=CARTESIAN_POINT ( 'NONE',  ( -18.30650389616927498, 59.06684029410003234, -4.447567583327522556 ) ) ;
#5155=CARTESIAN_POINT ( 'NONE',  ( -12.78406828249000782, 59.99816190035672747, -3.834978693179208697 ) ) ;
#5157=VERTEX_POINT ( 'NONE', #3380 ) ;
#5159=CIRCLE ( 'NONE', #20737, 5.999999999999998224 ) ;
#5162=CARTESIAN_POINT ( 'NONE',  ( -28.94833220779161920, 56.54499750659159929, -0.09259939256140287123 ) ) ;
#5189=CARTESIAN_POINT ( 'NONE',  ( 30.10683012259193703, 0.000000000000000000, -5.999999999999998224 ) ) ;
#5195=CARTESIAN_POINT ( 'NONE',  ( -14.12934535402923153, 71.18264261159711737, -4.639596491434939907 ) ) ;
#5205=EDGE_CURVE ( 'NONE', #9631, #19907, #2734, .T. ) ;
#5209=DIRECTION ( 'NONE',  ( 0.000000000000000000, -1.000000000000000000, 0.000000000000000000 ) ) ;
#5218=CARTESIAN_POINT ( 'NONE',  ( -11.87870293693008250, 79.99650906190652222, -12.16257741986773055 ) ) ;
#5227=CARTESIAN_POINT ( 'NONE',  ( -29.99999999999999645, 5.000000000000000888, 2.347807969642663029 ) ) ;
#5236=CARTESIAN_POINT ( 'NONE',  ( 1.499462569501769815, 53.04219685298476605, -3.436763594309801384 ) ) ;
#5237=CARTESIAN_POINT ( 'NONE',  ( 1.399080956625346150, 76.99412170571200420, -3.489245206103287256 ) ) ;
#5247=DIRECTION ( 'NONE',  ( 0.000000000000000000, 0.000000000000000000, 1.000000000000000000 ) ) ;
#5250=DIRECTION ( 'NONE',  ( 0.000000000000000000, 0.000000000000000000, -1.000000000000000000 ) ) ;
#5252=DIRECTION ( 'NONE',  ( 0.000000000000000000, 0.000000000000000000, 1.000000000000000000 ) ) ;
#5253=ORIENTED_EDGE ( 'NONE', *, *, #16935, .F. ) ;
#5257=ADVANCED_FACE ( 'NONE', ( #12302 ), #19644, .F. ) ;
#5264=CARTESIAN_POINT ( 'NONE',  ( -33.23999054399477160, 55.56111691158302790, -0.8200133748984262949 ) ) ;
#5265=CARTESIAN_POINT ( 'NONE',  ( -15.99999999999999289, 20.09941697557067997, 12.50000000000000000 ) ) ;
#5287=LINE ( 'NONE', #8693, #13640 ) ;
#5293=CARTESIAN_POINT ( 'NONE',  ( -15.99999999999999289, 80.00000000000000000, 0.000000000000000000 ) ) ;
#5296=CARTESIAN_POINT ( 'NONE',  ( -11.68625644715183931, 65.74999999999995737, -2.528164662410434804 ) ) ;
#5309=ADVANCED_FACE ( 'NONE', ( #11871, #18334, #2542 ), #947, .F. ) ;
#5315=CARTESIAN_POINT ( 'NONE',  ( 30.00000000000000000, 0.000000000000000000, 15.00000000000000000 ) ) ;
#5316=EDGE_CURVE ( 'NONE', #5484, #20070, #15074, .T. ) ;
#5321=CARTESIAN_POINT ( 'NONE',  ( -4.019148893687301438, 80.00000000016062529, -3.582299587995576573 ) ) ;
#5323=DIRECTION ( 'NONE',  ( -0.000000000000000000, -1.000000000000000000, -0.000000000000000000 ) ) ;
#5325=CARTESIAN_POINT ( 'NONE',  ( -32.66093446721252747, 78.07057667199779871, -5.137872117311673925 ) ) ;
#5328=CARTESIAN_POINT ( 'NONE',  ( -27.93274434770766135, 6.474012523638976724, 3.820265228604878605 ) ) ;
#5330=ORIENTED_EDGE ( 'NONE', *, *, #16935, .T. ) ;
#5337=CARTESIAN_POINT ( 'NONE',  ( -4.511339306326391352, 60.05354679878421109, 4.930296734904765721 ) ) ;
#5356=ORIENTED_EDGE ( 'NONE', *, *, #5004, .F. ) ;
#5366=CARTESIAN_POINT ( 'NONE',  ( -33.48120423251649669, 52.62637900463001728, -3.990501944831340353 ) ) ;
#5367=CARTESIAN_POINT ( 'NONE',  ( -17.62170904672685978, 19.84043322078894889, 12.39812820015802686 ) ) ;
#5389=DIRECTION ( 'NONE',  ( 0.000000000000000000, 0.000000000000000000, 1.000000000000000000 ) ) ;
#5391=DIRECTION ( 'NONE',  ( -0.000000000000000000, -0.000000000000000000, 1.000000000000000000 ) ) ;
#5393=DIRECTION ( 'NONE',  ( 0.000000000000000000, 0.000000000000000000, -1.000000000000000000 ) ) ;
#5394=CARTESIAN_POINT ( 'NONE',  ( -28.94340094228533644, 73.00589460461614522, 0.1996236911382455459 ) ) ;
#5403=ORIENTED_EDGE ( 'NONE', *, *, #10799, .T. ) ;
#5409=DIRECTION ( 'NONE',  ( 0.000000000000000000, -1.000000000000000000, 0.000000000000000000 ) ) ;
#5412=CARTESIAN_POINT ( 'NONE',  ( -20.08622074598449458, 79.99311222855624237, -11.99929078098927526 ) ) ;
#5413=DIRECTION ( 'NONE',  ( -1.000000000000000000, 0.000000000000000000, 0.000000000000000000 ) ) ;
#5417=( BOUNDED_SURFACE ( )  B_SPLINE_SURFACE ( 3, 2, ( 
 ( #18855, #19167, #4226 ),
 ( #17261, #20534, #14098 ),
 ( #1160, #20746, #9393 ),
 ( #10673, #2746, #17373 ),
 ( #9188, #15694, #6006 ),
 ( #12496, #7710, #18955 ),
 ( #14207, #20636, #6109 ),
 ( #12605, #19067, #11007 ),
 ( #15890, #12918, #8011 ),
 ( #13404, #11707, #19753 ),
 ( #477, #575, #18173 ),
 ( #5321, #11922, #16692 ),
 ( #12814, #10197, #11215 ),
 ( #17689, #15120, #2170 ),
 ( #8621, #16102, #1673 ),
 ( #14522, #16002, #19933 ),
 ( #3741, #7912, #8113 ),
 ( #14628, #7025, #373 ),
 ( #18385, #14412, #6818 ),
 ( #20841, #17784, #3638 ),
 ( #8519, #9707, #5424 ),
 ( #3156, #9606, #10089 ),
 ( #15018, #19853, #13512 ),
 ( #6418, #19958, #11810 ),
 ( #1465, #3252, #9501 ),
 ( #19271, #1568, #5218 ),
 ( #6317, #11318, #19371 ),
 ( #16579, #18272, #16199 ),
 ( #13304, #4844, #6919 ),
 ( #4740, #2064, #12025 ),
 ( #20383, #2270, #15641 ),
 ( #890, #788, #8935 ),
 ( #20174, #10517, #10731 ),
 ( #20073, #1108, #17211 ) ),
 .UNSPECIFIED., .F., .F., .T. ) 
 B_SPLINE_SURFACE_WITH_KNOTS ( ( 4, 2, 2, 2, 2, 2, 2, 2, 2, 2, 2, 2, 2, 2, 2, 2, 4 ),
 ( 3, 3 ),
 ( 0.01278509310405297195, 0.01434830319407976937, 0.01591151328410656679, 0.01669311832911996724, 0.01747472337413336421, 0.01903793346416016163, 0.02060114355418695906, 0.02216435364421375648, 0.02529077382426735479, 0.02685398391429415221, 0.02841719400432095310, 0.03154361418437454795, 0.03310682427440134190, 0.03467003436442814279, 0.03623324445445494368, 0.03701484949946834413, 0.03779645454448173764 ),
 ( 0.000000000000000000, 1.000000000000000000 ),
 .UNSPECIFIED. ) 
 GEOMETRIC_REPRESENTATION_ITEM ( )  RATIONAL_B_SPLINE_SURFACE ( (
 ( 1.000000000000000000, 0.7167790485004654766, 1.000000000000000000),
 ( 1.000000000000000000, 0.7293845257054283326, 1.000000000000000000),
 ( 1.000000000000000000, 0.7423068803280219452, 1.000000000000000000),
 ( 1.000000000000000000, 0.7686138469777443749, 1.000000000000000000),
 ( 1.000000000000000000, 0.7816781719487659874, 1.000000000000000000),
 ( 1.000000000000000000, 0.8009424076555987648, 1.000000000000000000),
 ( 1.000000000000000000, 0.8073105603346681924, 1.000000000000000000),
 ( 1.000000000000000000, 0.8199112611633488923, 1.000000000000000000),
 ( 1.000000000000000000, 0.8261570471473095312, 1.000000000000000000),
 ( 1.000000000000000000, 0.8443914605100146797, 1.000000000000000000),
 ( 1.000000000000000000, 0.8559617003904390620, 1.000000000000000000),
 ( 1.000000000000000000, 0.8778584927322264919, 1.000000000000000000),
 ( 1.000000000000000000, 0.8881844774554628064, 1.000000000000000000),
 ( 1.000000000000000000, 0.9075144288648415714, 1.000000000000000000),
 ( 1.000000000000000000, 0.9165151951639417538, 1.000000000000000000),
 ( 1.000000000000000000, 0.9409273377065782151, 1.000000000000000000),
 ( 1.000000000000000000, 0.9539926103733148421, 1.000000000000000000),
 ( 1.000000000000000000, 0.9694264545132288413, 1.000000000000000000),
 ( 1.000000000000000000, 0.9738877056526868969, 1.000000000000000000),
 ( 1.000000000000000000, 0.9815112523103146636, 1.000000000000000000),
 ( 1.000000000000000000, 0.9846522094487469845, 1.000000000000000000),
 ( 1.000000000000000000, 0.9924326897349095011, 1.000000000000000000),
 ( 1.000000000000000000, 0.9954310229819317568, 1.000000000000000000),
 ( 1.000000000000000000, 0.9981072485120819904, 1.000000000000000000),
 ( 1.000000000000000000, 0.9986952519232751291, 1.000000000000000000),
 ( 1.000000000000000000, 0.9994860253291516505, 1.000000000000000000),
 ( 1.000000000000000000, 0.9996937099786900038, 1.000000000000000000),
 ( 1.000000000000000000, 0.9999366964164366767, 1.000000000000000000),
 ( 1.000000000000000000, 0.9999724247964512092, 1.000000000000000000),
 ( 1.000000000000000000, 0.9999959980224297773, 1.000000000000000000),
 ( 1.000000000000000000, 0.9999982534776523657, 1.000000000000000000),
 ( 1.000000000000000000, 1.000000247701407607, 1.000000000000000000),
 ( 1.000000000000000000, 1.000000000000000000, 1.000000000000000000),
 ( 1.000000000000000000, 1.000000000000000000, 1.000000000000000000) ) ) 
 REPRESENTATION_ITEM ( '' )  SURFACE ( )  );
#5421=AXIS2_PLACEMENT_3D ( 'NONE', #16406, #12812, #8329 ) ;
#5424=CARTESIAN_POINT ( 'NONE',  ( -6.567413104170348070, 79.88387937455904364, -10.62823034224189556 ) ) ;
#5432=CARTESIAN_POINT ( 'NONE',  ( -29.99999999999999645, 5.000000000000000000, 10.11936314359214606 ) ) ;
#5442=CARTESIAN_POINT ( 'NONE',  ( 0.4495246258101979753, 59.24330822791731777, 1.356054076072180425 ) ) ;
#5453=AXIS2_PLACEMENT_3D ( 'NONE', #13516, #20078, #3745 ) ;
#5463=CARTESIAN_POINT ( 'NONE',  ( -14.99999999999999645, 0.000000000000000000, 15.00000000000000000 ) ) ;
#5474=CARTESIAN_POINT ( 'NONE',  ( -28.01889434176855431, 52.37691837744655743, -4.370015612845434383 ) ) ;
#5481=ORIENTED_EDGE ( 'NONE', *, *, #9926, .F. ) ;
#5484=VERTEX_POINT ( 'NONE', #9192 ) ;
#5490=VECTOR ( 'NONE', #19348, 1000.000000000000000 ) ;
#5493=CIRCLE ( 'NONE', #2875, 14.99999999999999645 ) ;
#5494=EDGE_CURVE ( 'NONE', #6871, #9039, #14317, .T. ) ;
#5499=CARTESIAN_POINT ( 'NONE',  ( -15.99999999999999289, 15.09941697557068530, 0.9999999999999991118 ) ) ;
#5510=CARTESIAN_POINT ( 'NONE',  ( -3.049535234737931866, 65.74999999999998579, 3.381771649840966010 ) ) ;
#5512=CARTESIAN_POINT ( 'NONE',  ( -29.99999999999999645, 5.000000000000000000, 15.00000000000000000 ) ) ;
#5515=ORIENTED_EDGE ( 'NONE', *, *, #5834, .F. ) ;
#5524=CARTESIAN_POINT ( 'NONE',  ( -25.43258689582962973, 79.88387937455904364, -10.62823034224189911 ) ) ;
#5536=DIRECTION ( 'NONE',  ( 0.000000000000000000, 0.000000000000000000, -1.000000000000000000 ) ) ;
#5553=CARTESIAN_POINT ( 'NONE',  ( 30.10683012259193703, 5.000000000000000000, 0.000000000000000000 ) ) ;
#5554=CARTESIAN_POINT ( 'NONE',  ( -35.00000000000000000, 64.25000000000000000, 1.479896280015796650 ) ) ;
#5555=DIRECTION ( 'NONE',  ( 0.000000000000000000, 0.000000000000000000, -1.000000000000000000 ) ) ;
#5577=CARTESIAN_POINT ( 'NONE',  ( -24.74148270909007152, 49.98498879254805161, -8.950542976129836958 ) ) ;
#5581=CARTESIAN_POINT ( 'NONE',  ( -27.90532276960012936, 55.94151689669796923, 3.821265830397637231 ) ) ;
#5595=B_SPLINE_CURVE_WITH_KNOTS ( 'NONE', 3,
 ( #7044, #2289, #7151, #4298 ),
 .UNSPECIFIED., .F., .F.,
 ( 4, 4 ),
 ( 0.000000000000000000, 0.001416029653785004505 ),
 .UNSPECIFIED. ) ;
#5597=DIRECTION ( 'NONE',  ( 1.000000000000000000, -0.000000000000000000, -0.000000000000000000 ) ) ;
#5598=CARTESIAN_POINT ( 'NONE',  ( -14.69197289804462159, 19.93670296710511636, 12.43566393466945108 ) ) ;
#5604=VECTOR ( 'NONE', #7997, 1000.000000000000000 ) ;
#5606=CARTESIAN_POINT ( 'NONE',  ( -28.12331899344885500, 75.90505089108978609, 3.056606027158062400 ) ) ;
#5626=CARTESIAN_POINT ( 'NONE',  ( -11.09026189855725164, 15.09941697557061957, 0.9457651797582804498 ) ) ;
#5647=CARTESIAN_POINT ( 'NONE',  ( -29.99999999999999645, 5.000000000000000888, 3.748555621732009069 ) ) ;
#5655=AXIS2_PLACEMENT_3D ( 'NONE', #5553, #12043, #3980 ) ;
#5659=DIRECTION ( 'NONE',  ( 1.000000000000000000, 0.000000000000000000, -1.224646799147353207E-16 ) ) ;
#5669=AXIS2_PLACEMENT_3D ( 'NONE', #16802, #686, #15848 ) ;
#5672=PRODUCT ( 'Base Lock Knob', 'Base Lock Knob', '', ( #2781 ) ) ;
#5676=CARTESIAN_POINT ( 'NONE',  ( -16.18016922445852046, 71.61437827766147279, -4.999999999999992895 ) ) ;
#5681=CARTESIAN_POINT ( 'NONE',  ( -27.50943688352612782, 50.00306753912056479, -13.03837235451981336 ) ) ;
#5685=EDGE_LOOP ( 'NONE', ( #18408, #2649, #17236 ) ) ;
#5702=CARTESIAN_POINT ( 'NONE',  ( -11.66788315198026638, 17.61676080837512970, 11.72685522487003951 ) ) ;
#5713=CARTESIAN_POINT ( 'NONE',  ( -0.1767699604045824824, 65.74999999999997158, 2.481238266578629226 ) ) ;
#5729=ADVANCED_FACE ( 'NONE', ( #3125 ), #14284, .T. ) ;
#5730=CARTESIAN_POINT ( 'NONE',  ( 44.00000000000000000, 0.000000000000000000, -15.00000000000000355 ) ) ;
#5746=CARTESIAN_POINT ( 'NONE',  ( -16.93678575793154550, 80.00001702024998451, -12.48679740715397379 ) ) ;
#5760=LINE ( 'NONE', #6459, #10507 ) ;
#5770=ORIENTED_EDGE ( 'NONE', *, *, #2675, .F. ) ;
#5776=EDGE_LOOP ( 'NONE', ( #7416, #1022, #12887, #14631 ) ) ;
#5786=ORIENTED_EDGE ( 'NONE', *, *, #13010, .F. ) ;
#5791=CARTESIAN_POINT ( 'NONE',  ( -24.31754996354614207, 49.87382451390904237, -9.352669984570907147 ) ) ;
#5795=CIRCLE ( 'NONE', #12254, 4.999999999999995559 ) ;
#5796=DIRECTION ( 'NONE',  ( 1.000000000000000000, 0.000000000000000000, 0.000000000000000000 ) ) ;
#5803=VERTEX_POINT ( 'NONE', #6187 ) ;
#5806=CARTESIAN_POINT ( 'NONE',  ( 1.425125561529466012, 54.47798152960064755, -1.780651232228821046 ) ) ;
#5810=DIRECTION ( 'NONE',  ( -0.000000000000000000, 1.000000000000000000, -0.000000000000000000 ) ) ;
#5817=DIRECTION ( 'NONE',  ( 0.000000000000000000, -0.000000000000000000, 1.000000000000000000 ) ) ;
#5834=EDGE_CURVE ( 'NONE', #6959, #13646, #10877, .T. ) ;
#5838=CARTESIAN_POINT ( 'NONE',  ( 45.00000000000000000, -10.00000000000000000, -15.00000000000000000 ) ) ;
#5840=FACE_BOUND ( 'NONE', #15435, .T. ) ;
#5848=ORIENTED_EDGE ( 'NONE', *, *, #7327, .F. ) ;
#5849=CARTESIAN_POINT ( 'NONE',  ( -3.649238679178553380, 77.92717739396518084, 2.017250382391169605 ) ) ;
#5853=EDGE_CURVE ( 'NONE', #3287, #4912, #407, .T. ) ;
#5855=ORIENTED_EDGE ( 'NONE', *, *, #17705, .T. ) ;
#5860=CARTESIAN_POINT ( 'NONE',  ( -35.00000000000000000, 64.25000000000000000, -1.525597966176003961 ) ) ;
#5870=DIRECTION ( 'NONE',  ( 0.000000000000000000, -1.000000000000000000, 0.000000000000000000 ) ) ;
#5871=CARTESIAN_POINT ( 'NONE',  ( -4.705817999896520831, 64.80165467510407495, 5.356440324370162820 ) ) ;
#5875=FACE_OUTER_BOUND ( 'NONE', #711, .T. ) ;
#5891=CARTESIAN_POINT ( 'NONE',  ( -22.79285140204124716, 49.64535697708226536, -10.50220247801678752 ) ) ;
#5902=EDGE_LOOP ( 'NONE', ( #18095, #16975, #745, #16401 ) ) ;
#5905=CARTESIAN_POINT ( 'NONE',  ( -32.78929790297351587, 51.06562928705771753, -6.895168070231495250 ) ) ;
#5911=ORIENTED_EDGE ( 'NONE', *, *, #10029, .F. ) ;
#5916=CARTESIAN_POINT ( 'NONE',  ( -11.16353062760892634, 16.40948116617020958, 11.52664465621722734 ) ) ;
#5923=DIRECTION ( 'NONE',  ( 0.000000000000000000, -1.000000000000000000, 0.000000000000000000 ) ) ;
#5925=CARTESIAN_POINT ( 'NONE',  ( -11.59722103597593801, 11.66854079980773129, 3.430876175762954006 ) ) ;
#5930=AXIS2_PLACEMENT_3D ( 'NONE', #17098, #16989, #4478 ) ;
#5932=CARTESIAN_POINT ( 'NONE',  ( -0.1767699604045824824, 64.25000000000000000, 2.481238266578627449 ) ) ;
#5937=FACE_OUTER_BOUND ( 'NONE', #12258, .T. ) ;
#5961=ORIENTED_EDGE ( 'NONE', *, *, #5316, .F. ) ;
#5970=EDGE_CURVE ( 'NONE', #4222, #11795, #3131, .T. ) ;
#5977=CYLINDRICAL_SURFACE ( 'NONE', #1693, 5.999999999999998224 ) ;
#5979=ORIENTED_EDGE ( 'NONE', *, *, #2807, .F. ) ;
#5988=LINE ( 'NONE', #4722, #18556 ) ;
#5989=ORIENTED_EDGE ( 'NONE', *, *, #1391, .T. ) ;
#5995=CARTESIAN_POINT ( 'NONE',  ( -22.24814625259552869, 45.17694441447353881, -10.83184487622254899 ) ) ;
#5998=CARTESIAN_POINT ( 'NONE',  ( -27.50045467171848301, 45.80088190002059889, -4.911061130343635561 ) ) ;
#6006=CARTESIAN_POINT ( 'NONE',  ( 1.204513484672493639, 77.44204738084411588, -4.113378397035853062 ) ) ;
#6009=DIRECTION ( 'NONE',  ( 0.000000000000000000, 0.000000000000000000, -1.000000000000000000 ) ) ;
#6011=CARTESIAN_POINT ( 'NONE',  ( -33.40960586970430768, 54.51484073799145591, -1.766275756695815380 ) ) ;
#6012=CARTESIAN_POINT ( 'NONE',  ( -27.39744768730504987, 9.624020198635008683, 5.177064134126243111 ) ) ;
#6017=ORIENTED_EDGE ( 'NONE', *, *, #17179, .T. ) ;
#6020=AXIS2_PLACEMENT_3D ( 'NONE', #3095, #15929, #6248 ) ;
#6025=( GEOMETRIC_REPRESENTATION_CONTEXT ( 3 ) GLOBAL_UNCERTAINTY_ASSIGNED_CONTEXT ( ( #8277 ) ) GLOBAL_UNIT_ASSIGNED_CONTEXT ( ( #15806, #4550, #11229 ) ) REPRESENTATION_CONTEXT ( 'NONE', 'WORKASPACE' ) );
#6026=DIRECTION ( 'NONE',  ( -1.000000000000000000, -0.000000000000000000, -0.000000000000000000 ) ) ;
#6040=CARTESIAN_POINT ( 'NONE',  ( -3.541693527980152023, 79.08610913872911397, 1.260722419662599236 ) ) ;
#6042=SHAPE_DEFINITION_REPRESENTATION ( #9067, #3951 ) ;
#6072=FACE_OUTER_BOUND ( 'NONE', #2848, .T. ) ;
#6073=VECTOR ( 'NONE', #3626, 1000.000000000000000 ) ;
#6075=CARTESIAN_POINT ( 'NONE',  ( -15.99999999999999289, 0.000000000000000000, 0.000000000000000000 ) ) ;
#6077=AXIS2_PLACEMENT_3D ( 'NONE', #7257, #5659, #18611 ) ;
#6078=CYLINDRICAL_SURFACE ( 'NONE', #329, 13.99999999999999822 ) ;
#6088=DIRECTION ( 'NONE',  ( 1.000000000000000000, -0.000000000000000000, -0.000000000000000000 ) ) ;
#6089=FACE_OUTER_BOUND ( 'NONE', #2679, .T. ) ;
#6099=CARTESIAN_POINT ( 'NONE',  ( -5.772503121411054039, 50.66968791804065830, -7.229964842171530570 ) ) ;
#6103=CARTESIAN_POINT ( 'NONE',  ( -19.05307565254539526, 45.50731414553807497, -12.12761656432236279 ) ) ;
#6109=CARTESIAN_POINT ( 'NONE',  ( 0.8940010539731342298, 77.84073441274544791, -4.744404894158055441 ) ) ;
#6110=CIRCLE ( 'NONE', #18645, 5.999999999999998224 ) ;
#6112=EDGE_LOOP ( 'NONE', ( #3721, #554, #4698, #13492, #4436, #5481, #16637, #11954 ) ) ;
#6115=CARTESIAN_POINT ( 'NONE',  ( -33.44495115927801976, 54.23679612179412146, -2.044894016340141896 ) ) ;
#6117=ORIENTED_EDGE ( 'NONE', *, *, #16814, .T. ) ;
#6124=CIRCLE ( 'NONE', #8162, 5.999999999999998224 ) ;
#6134=CARTESIAN_POINT ( 'NONE',  ( -19.76533548850507316, 18.40525104484276397, 11.92183032960170586 ) ) ;
#6136=CARTESIAN_POINT ( 'NONE',  ( -31.93815604754423632, 67.52062497874923963, 2.295552037966095416 ) ) ;
#6144=DIRECTION ( 'NONE',  ( 1.000000000000000000, 0.000000000000000000, 0.000000000000000000 ) ) ;
#6149=ORIENTED_EDGE ( 'NONE', *, *, #868, .F. ) ;
#6156=CARTESIAN_POINT ( 'NONE',  ( 0.1080579935186935236, 61.16269310544473825, 2.006079461162327160 ) ) ;
#6159=CARTESIAN_POINT ( 'NONE',  ( -15.99999999999999289, 15.09941697557068530, 0.9999999999999991118 ) ) ;
#6172=CARTESIAN_POINT ( 'NONE',  ( -33.50112344255473573, 76.50873768553087473, -2.871813542385711848 ) ) ;
#6175=( NAMED_UNIT ( * ) PLANE_ANGLE_UNIT ( ) SI_UNIT ( $, .RADIAN. ) );
#6176=PRODUCT_DEFINITION_CONTEXT ( 'detailed design', #6880, 'design' ) ;
#6186=EDGE_LOOP ( 'NONE', ( #9589, #20225, #8142 ) ) ;
#6187=CARTESIAN_POINT ( 'NONE',  ( 44.00000000000000000, 0.000000000000000000, -15.00000000000000355 ) ) ;
#6192=VERTEX_POINT ( 'NONE', #17522 ) ;
#6206=CARTESIAN_POINT ( 'NONE',  ( -1.904422244483446214, 50.06947204901834425, -10.93639821325584016 ) ) ;
#6209=CARTESIAN_POINT ( 'NONE',  ( -23.85050882933249738, 45.02920876159776498, -9.734908535650388828 ) ) ;
#6213=DIRECTION ( 'NONE',  ( 1.000000000000000000, 0.000000000000000000, 0.000000000000000000 ) ) ;
#6216=ORIENTED_EDGE ( 'NONE', *, *, #5494, .F. ) ;
#6221=CARTESIAN_POINT ( 'NONE',  ( -9.814647292144057289, 50.28451303171664222, -15.41809052414373049 ) ) ;
#6237=CARTESIAN_POINT ( 'NONE',  ( -15.99999999999999289, 10.09941697557069418, 4.999999999999989342 ) ) ;
#6243=CARTESIAN_POINT ( 'NONE',  ( -0.06184395245637178823, 67.52062497875388658, 2.295552037965487013 ) ) ;
#6248=DIRECTION ( 'NONE',  ( 0.000000000000000000, 0.000000000000000000, 1.000000000000000000 ) ) ;
#6255=EDGE_CURVE ( 'NONE', #4315, #14773, #19719, .T. ) ;
#6258=CIRCLE ( 'NONE', #18811, 12.50000000000000000 ) ;
#6259=CARTESIAN_POINT ( 'NONE',  ( -11.10102051443364779, 16.09941697557071905, 0.9999999999999997780 ) ) ;
#6260=EDGE_LOOP ( 'NONE', ( #17951, #10716, #7342, #11741 ) ) ;
#6266=DIRECTION ( 'NONE',  ( 0.000000000000000000, 0.000000000000000000, -1.000000000000000000 ) ) ;
#6272=PLANE ( 'NONE',  #11247 ) ;
#6278=CARTESIAN_POINT ( 'NONE',  ( -27.95202372264500212, 79.14876326484322533, -7.307758369671589094 ) ) ;
#6287=CIRCLE ( 'NONE', #20499, 5.000000000000000000 ) ;
#6289=CARTESIAN_POINT ( 'NONE',  ( 30.10683012259193703, 0.000000000000000000, 0.000000000000000000 ) ) ;
#6303=ORIENTED_EDGE ( 'NONE', *, *, #2153, .F. ) ;
#6306=CARTESIAN_POINT ( 'NONE',  ( -5.637571478551725690, 50.76112637345350720, -7.048071971797520874 ) ) ;
#6313=ORIENTED_EDGE ( 'NONE', *, *, #14874, .F. ) ;
#6317=CARTESIAN_POINT ( 'NONE',  ( -12.43358389273065256, 79.99999999999585043, -11.99131545410286925 ) ) ;
#6318=ORIENTED_EDGE ( 'NONE', *, *, #309, .T. ) ;
#6322=CARTESIAN_POINT ( 'NONE',  ( -32.43274721513416381, 59.32595788850117202, 1.390757872376907178 ) ) ;
#6325=ORIENTED_EDGE ( 'NONE', *, *, #3839, .F. ) ;
#6326=CARTESIAN_POINT ( 'NONE',  ( -0.1286331481417117006, 66.76123571212174568, 2.404802591979303905 ) ) ;
#6332=CARTESIAN_POINT ( 'NONE',  ( -27.29754541467060491, 63.83810381476320828, 5.349348394099980197 ) ) ;
#6336=CARTESIAN_POINT ( 'NONE',  ( -27.38439717691917608, 68.36083330498577482, 5.162430512333705757 ) ) ;
#6344=CARTESIAN_POINT ( 'NONE',  ( -1.124748988296088825, 64.25000000000000000, 2.549678278787572250 ) ) ;
#6351=CARTESIAN_POINT ( 'NONE',  ( -20.89897948556633978, 14.09941697557065332, 0.9999999999999991118 ) ) ;
#6372=CARTESIAN_POINT ( 'NONE',  ( 45.00000000000000000, 5.000000000000000000, 15.00000000000000000 ) ) ;
#6379=CARTESIAN_POINT ( 'NONE',  ( -28.32806265867318984, 79.99999999995431210, -2.072940693967530557 ) ) ;
#6383=B_SPLINE_CURVE_WITH_KNOTS ( 'NONE', 3,
 ( #8858, #603, #13436, #12267 ),
 .UNSPECIFIED., .F., .F.,
 ( 4, 4 ),
 ( 0.000000000000000000, 0.001416029653785006890 ),
 .UNSPECIFIED. ) ;
#6400=CARTESIAN_POINT ( 'NONE',  ( -26.66531713196410891, 5.892095953840440714, -6.547001825740162317 ) ) ;
#6408=CARTESIAN_POINT ( 'NONE',  ( -1.117320739478655733, 50.20017401731518447, -10.03899822371341344 ) ) ;
#6415=CARTESIAN_POINT ( 'NONE',  ( -15.99999999999991651, 71.61437827766162911, -4.999999999999997335 ) ) ;
#6418=CARTESIAN_POINT ( 'NONE',  ( -10.55030972131536338, 80.00000000004204992, -11.26030642047042996 ) ) ;
#6424=CARTESIAN_POINT ( 'NONE',  ( -12.09679518933233311, 61.49126500257621331, -3.129598480498282598 ) ) ;
#6429=EDGE_CURVE ( 'NONE', #3253, #16503, #18354, .T. ) ;
#6434=CARTESIAN_POINT ( 'NONE',  ( -28.99999999999999289, 0.000000000000000000, -15.00000000000000000 ) ) ;
#6443=ORIENTED_EDGE ( 'NONE', *, *, #14431, .T. ) ;
#6448=CARTESIAN_POINT ( 'NONE',  ( -14.37945692259737207, 10.36644441490629909, 12.39552528635021034 ) ) ;
#6450=CARTESIAN_POINT ( 'NONE',  ( -18.33199948130959100, 79.99972521406444059, -12.39529528716347428 ) ) ;
#6454=FACE_OUTER_BOUND ( 'NONE', #659, .T. ) ;
#6459=CARTESIAN_POINT ( 'NONE',  ( 44.00000000000000000, 0.000000000000000000, -15.00000000000000355 ) ) ;
#6468=DIRECTION ( 'NONE',  ( 0.000000000000000000, 0.000000000000000000, -1.000000000000000000 ) ) ;
#6479=CARTESIAN_POINT ( 'NONE',  ( -32.41958609996412122, 70.63162242946638969, 1.437809060325973221 ) ) ;
#6482=CARTESIAN_POINT ( 'NONE',  ( -29.47154141322603138, 77.37584602520398391, -3.922623763563328314 ) ) ;
#6501=CARTESIAN_POINT ( 'NONE',  ( 0.000000000000000000, -10.00000000000000000, 0.000000000000000000 ) ) ;
#6503=LINE ( 'NONE', #13207, #9992 ) ;
#6504=CARTESIAN_POINT ( 'NONE',  ( -26.00000000000000000, 5.000000000000001776, -7.500000000000000000 ) ) ;
#6509=CIRCLE ( 'NONE', #9226, 17.50000000000000000 ) ;
#6513=CARTESIAN_POINT ( 'NONE',  ( -12.60528683216188739, 45.48061573273304958, -12.04982389388483632 ) ) ;
#6514=CARTESIAN_POINT ( 'NONE',  ( 1.237363539717748262, 77.39914922625320060, -4.045904646045205055 ) ) ;
#6515=ADVANCED_FACE ( 'NONE', ( #4563 ), #7410, .T. ) ;
#6517=CARTESIAN_POINT ( 'NONE',  ( -24.71655914096720608, 44.99675394863319866, -8.967748501840956621 ) ) ;
#6522=PLANE ( 'NONE',  #7127 ) ;
#6523=EDGE_CURVE ( 'NONE', #15273, #20835, #12195, .T. ) ;
#6525=CARTESIAN_POINT ( 'NONE',  ( -19.20871456446631598, 60.00315144574870629, -3.836613224171040670 ) ) ;
#6527=CARTESIAN_POINT ( 'NONE',  ( -31.83568508345510750, 63.85501752543220988, 2.461464410061926955 ) ) ;
#6549=DIRECTION ( 'NONE',  ( 0.000000000000000000, -1.000000000000000000, 0.000000000000000000 ) ) ;
#6560=CARTESIAN_POINT ( 'NONE',  ( -0.1517743604773433008, 63.45732323195518632, 2.441554792792626660 ) ) ;
#6570=EDGE_LOOP ( 'NONE', ( #9153, #3130, #8764, #16268, #15703 ) ) ;
#6574=CARTESIAN_POINT ( 'NONE',  ( -14.60189797479694818, 71.38521106151608819, -4.803508630518933842 ) ) ;
#6578=VERTEX_POINT ( 'NONE', #7522 ) ;
#6579=DIRECTION ( 'NONE',  ( 0.000000000000000000, 0.000000000000000000, -1.000000000000000000 ) ) ;
#6582=CARTESIAN_POINT ( 'NONE',  ( -33.48481952675158624, 76.25000000000001421, -2.578432583507804132 ) ) ;
#6585=CARTESIAN_POINT ( 'NONE',  ( -29.45159263616708500, 77.71408077849254425, -4.406821185033810373 ) ) ;
#6596=AXIS2_PLACEMENT_3D ( 'NONE', #16514, #13341, #19789 ) ;
#6597=FACE_OUTER_BOUND ( 'NONE', #1514, .T. ) ;
#6602=DIRECTION ( 'NONE',  ( 0.000000000000000000, 0.000000000000000000, -1.000000000000000000 ) ) ;
#6609=VERTEX_POINT ( 'NONE', #11628 ) ;
#6617=CARTESIAN_POINT ( 'NONE',  ( -4.201979992901475391, 56.88514657979481370, 4.132832673961413406 ) ) ;
#6618=CARTESIAN_POINT ( 'NONE',  ( -15.99999999999999289, 80.00000000000000000, 12.50000000000000000 ) ) ;
#6626=DIRECTION ( 'NONE',  ( 0.000000000000000000, 0.000000000000000000, -1.000000000000000000 ) ) ;
#6629=CARTESIAN_POINT ( 'NONE',  ( -18.90941040546627860, 59.62118480013949551, -4.068652614656587119 ) ) ;
#6632=CIRCLE ( 'NONE', #18504, 5.999999999999989342 ) ;
#6633=CARTESIAN_POINT ( 'NONE',  ( -15.64137421610944578, 58.39658375749213803, -4.990290896351837091 ) ) ;
#6635=ORIENTED_EDGE ( 'NONE', *, *, #10708, .T. ) ;
#6642=CARTESIAN_POINT ( 'NONE',  ( -27.29940250357268283, 45.63043474242538622, -5.355865623545788878 ) ) ;
#6649=B_SPLINE_CURVE_WITH_KNOTS ( 'NONE', 3,
 ( #15896, #2753, #18864, #4337, #12612, #2648, #9194, #9091, #7920, #12713, #9294, #15700, #14419, #1166, #4649, #4545, #12822, #3057, #14105, #7614, #6012, #12502, #18963, #4441 ),
 .UNSPECIFIED., .F., .F.,
 ( 4, 2, 2, 2, 2, 2, 2, 2, 2, 2, 2, 4 ),
 ( 0.000000000000000000, 0.002039071642891474370, 0.003058607464337211555, 0.004078143285782949608, 0.006117214928674423111, 0.007136750750120161163, 0.008156286571565897481, 0.009175822393011635533, 0.01019535821445737185, 0.01223442985734884796, 0.01427350150024032753, 0.01631257314313180537 ),
 .UNSPECIFIED. ) ;
#6654=EDGE_CURVE ( 'NONE', #17576, #14829, #17711, .T. ) ;
#6659=DIRECTION ( 'NONE',  ( 0.000000000000000000, -1.000000000000000000, 0.000000000000000000 ) ) ;
#6668=ORIENTED_EDGE ( 'NONE', *, *, #11825, .T. ) ;
#6704=AXIS2_PLACEMENT_3D ( 'NONE', #15947, #4796, #4594 ) ;
#6709=CARTESIAN_POINT ( 'NONE',  ( -27.12730151730438521, 6.201679376448834269, -5.736216294243367209 ) ) ;
#6710=SHAPE_REPRESENTATION_RELATIONSHIP ( 'NONE' , 'NONE' ,  #3951, #15173 ) ;
#6714=CARTESIAN_POINT ( 'NONE',  ( -4.701390418375632763, 64.25000000000000000, 5.347094680480811490 ) ) ;
#6718=CARTESIAN_POINT ( 'NONE',  ( -3.770603668498050176, 53.17095540632753625, 2.595721307129207567 ) ) ;
#6724=ORIENTED_EDGE ( 'NONE', *, *, #12734, .F. ) ;
#6727=VERTEX_POINT ( 'NONE', #14542 ) ;
#6729=CYLINDRICAL_SURFACE ( 'NONE', #9828, 14.99999999999999645 ) ;
#6737=ORIENTED_EDGE ( 'NONE', *, *, #18496, .F. ) ;
#6746=CARTESIAN_POINT ( 'NONE',  ( -28.38754368462288369, 47.74392439351031214, -1.698457930398967308 ) ) ;
#6749=VERTEX_POINT ( 'NONE', #6842 ) ;
#6750=FACE_OUTER_BOUND ( 'NONE', #8886, .T. ) ;
#6764=CARTESIAN_POINT ( 'NONE',  ( -28.22805963754889191, 65.74999999999998579, 3.997049355788913960 ) ) ;
#6765=EDGE_CURVE ( 'NONE', #17780, #3281, #11969, .T. ) ;
#6775=ORIENTED_EDGE ( 'NONE', *, *, #8345, .T. ) ;
#6786=CARTESIAN_POINT ( 'NONE',  ( -13.42979308546154193, 70.72677659407449369, -4.297493274131825913 ) ) ;
#6787=AXIS2_PLACEMENT_3D ( 'NONE', #19512, #133, #16353 ) ;
#6802=CARTESIAN_POINT ( 'NONE',  ( -17.04221037121256899, 79.99997668367075221, -12.46941917154160961 ) ) ;
#6818=CARTESIAN_POINT ( 'NONE',  ( -5.239423594773973569, 79.79422864173673702, -10.01493943371665907 ) ) ;
#6820=STYLED_ITEM('',(#20967),#3293);
#6826=CARTESIAN_POINT ( 'NONE',  ( -32.29388722507494691, 78.35452279512254847, -5.666775083474093755 ) ) ;
#6831=EDGE_CURVE ( 'NONE', #2307, #11320, #5595, .T. ) ;
#6839=CARTESIAN_POINT ( 'NONE',  ( -4.055026664453261098, 55.59176219034431199, 3.696206164233441172 ) ) ;
#6840=CARTESIAN_POINT ( 'NONE',  ( -5.615923431034060442, 79.82407219761680039, -10.19945363082080902 ) ) ;
#6842=CARTESIAN_POINT ( 'NONE',  ( -15.99999999999999289, 4.999999999999997335, -17.50000000000000000 ) ) ;
#6856=FACE_OUTER_BOUND ( 'NONE', #1530, .T. ) ;
#6857=DIRECTION ( 'NONE',  ( 0.000000000000000000, 0.000000000000000000, 1.000000000000000000 ) ) ;
#6858=VECTOR ( 'NONE', #20656, 1000.000000000000000 ) ;
#6863=CARTESIAN_POINT ( 'NONE',  ( -28.50825147543515214, 49.06444853241422521, -0.2686478949330403654 ) ) ;
#6871=VERTEX_POINT ( 'NONE', #4192 ) ;
#6872=CARTESIAN_POINT ( 'NONE',  ( -3.348702641817554060, 65.53858748455307648, 2.490407514064874039 ) ) ;
#6880=APPLICATION_CONTEXT ( 'automotive_design' ) ;
#6903=ORIENTED_EDGE ( 'NONE', *, *, #9402, .F. ) ;
#6905=CARTESIAN_POINT ( 'NONE',  ( -15.99999999999999289, 79.99999999999998579, -12.50000000000000000 ) ) ;
#6916=CARTESIAN_POINT ( 'NONE',  ( 10.49211908931699178, 0.000000000000000000, 0.000000000000000000 ) ) ;
#6919=CARTESIAN_POINT ( 'NONE',  ( -13.92188866561930993, 79.99981534483862333, -12.41883285859719344 ) ) ;
#6924=EDGE_CURVE ( 'NONE', #5803, #17269, #5760, .T. ) ;
#6927=CARTESIAN_POINT ( 'NONE',  ( -29.99999999999993605, 5.000000000000018652, 8.518881768062307458 ) ) ;
#6930=EDGE_CURVE ( 'NONE', #7189, #17545, #1718, .T. ) ;
#6932=CARTESIAN_POINT ( 'NONE',  ( -3.659121735415404864, 47.49494768642473730, -2.010530405749917371 ) ) ;
#6935=CARTESIAN_POINT ( 'NONE',  ( -3.123205458604330076, 58.78078776664096239, 1.164416042648590777 ) ) ;
#6936=CARTESIAN_POINT ( 'NONE',  ( 1.484819526751601559, 76.25000000000000000, -2.578432583507792142 ) ) ;
#6946=TOROIDAL_SURFACE ( 'NONE', #3579, 17.50000000000000000, 5.000000000000000000 ) ;
#6949=CARTESIAN_POINT ( 'NONE',  ( -11.68625644715183931, 64.25000000000000000, -2.528164662410438357 ) ) ;
#6959=VERTEX_POINT ( 'NONE', #9652 ) ;
#6963=EDGE_CURVE ( 'NONE', #13750, #4880, #13955, .T. ) ;
#6965=CARTESIAN_POINT ( 'NONE',  ( -32.68402340442658982, 50.97242918334629280, -7.141224787959053799 ) ) ;
#6971=ORIENTED_EDGE ( 'NONE', *, *, #14731, .F. ) ;
#6972=AXIS2_PLACEMENT_3D ( 'NONE', #19940, #5409, #16772 ) ;
#6981=ORIENTED_EDGE ( 'NONE', *, *, #10160, .F. ) ;
#6984=VERTEX_POINT ( 'NONE', #9551 ) ;
#6988=ORIENTED_EDGE ( 'NONE', *, *, #15224, .T. ) ;
#6990=CARTESIAN_POINT ( 'NONE',  ( -29.99999999999999645, 5.000000000000000000, 15.00000000000000000 ) ) ;
#6998=CARTESIAN_POINT ( 'NONE',  ( -4.239935945710826104, 64.25000000000000000, 4.526879896143025661 ) ) ;
#7011=CARTESIAN_POINT ( 'NONE',  ( -23.54107059693361492, 80.00000000014368595, -10.01181548797457488 ) ) ;
#7012=CARTESIAN_POINT ( 'NONE',  ( 0.000000000000000000, -10.00000000000000000, -30.00000000000000000 ) ) ;
#7024=DIRECTION ( 'NONE',  ( 0.000000000000000000, 0.000000000000000000, -1.000000000000000000 ) ) ;
#7025=CARTESIAN_POINT ( 'NONE',  ( -5.550616763087108829, 79.57013539180735506, -8.777265990090908687 ) ) ;
#7026=EDGE_CURVE ( 'NONE', #9010, #17344, #18301, .T. ) ;
#7043=ORIENTED_EDGE ( 'NONE', *, *, #8345, .F. ) ;
#7044=CARTESIAN_POINT ( 'NONE',  ( 26.99999999999999645, 65.74999999999995737, -2.528164662410434804 ) ) ;
#7045=CARTESIAN_POINT ( 'NONE',  ( -3.575197966166810737, 53.09951303229428987, -3.365123708265559621 ) ) ;
#7062=CARTESIAN_POINT ( 'NONE',  ( -35.00000000000000000, 64.25000000000000000, 1.479896280015796650 ) ) ;
#7072=CARTESIAN_POINT ( 'NONE',  ( -15.99999999999999289, 64.25000000000000000, 0.000000000000000000 ) ) ;
#7073=DIRECTION ( 'NONE',  ( 1.000000000000000000, 0.000000000000000000, 0.000000000000000000 ) ) ;
#7074=CARTESIAN_POINT ( 'NONE',  ( -26.27766216112225095, 45.15629102170652232, -7.122914202326710686 ) ) ;
#7086=ORIENTED_EDGE ( 'NONE', *, *, #2153, .T. ) ;
#7119=PLANE ( 'NONE',  #15142 ) ;
#7127=AXIS2_PLACEMENT_3D ( 'NONE', #1779, #19269, #6626 ) ;
#7134=ORIENTED_EDGE ( 'NONE', *, *, #19402, .F. ) ;
#7138=DIRECTION ( 'NONE',  ( 0.000000000000000000, 0.000000000000000000, -1.000000000000000000 ) ) ;
#7139=AXIS2_PLACEMENT_3D ( 'NONE', #14600, #17973, #17874 ) ;
#7141=CARTESIAN_POINT ( 'NONE',  ( -28.06876874214889384, 9.090108580520308124, 3.321481296491451740 ) ) ;
#7151=CARTESIAN_POINT ( 'NONE',  ( 27.66662763442663575, 65.75000000000001421, -1.859747928060466293 ) ) ;
#7164=AXIS2_PLACEMENT_3D ( 'NONE', #16652, #8691, #8999 ) ;
#7165=ORIENTED_EDGE ( 'NONE', *, *, #9087, .T. ) ;
#7180=CARTESIAN_POINT ( 'NONE',  ( -17.93384870776856133, 50.46031766474980884, -16.18952312236656255 ) ) ;
#7189=VERTEX_POINT ( 'NONE', #18136 ) ;
#7190=EDGE_CURVE ( 'NONE', #20014, #1893, #13164, .T. ) ;
#7195=ORIENTED_EDGE ( 'NONE', *, *, #7190, .F. ) ;
#7209=VECTOR ( 'NONE', #8027, 1000.000000000000000 ) ;
#7223=EDGE_LOOP ( 'NONE', ( #10410, #3210, #17222, #7383 ) ) ;
#7225=CARTESIAN_POINT ( 'NONE',  ( -21.44969027868145162, 80.00000000004207834, -11.26030642047179420 ) ) ;
#7232=CARTESIAN_POINT ( 'NONE',  ( 28.00000000000001066, 65.75000000000001421, 75.00000000000000000 ) ) ;
#7236=DIRECTION ( 'NONE',  ( -1.000000000000000000, 0.000000000000000000, 0.000000000000000000 ) ) ;
#7238=CARTESIAN_POINT ( 'NONE',  ( -15.99999999999999289, -10.00000000000000000, -5.999999999999989342 ) ) ;
#7245=CARTESIAN_POINT ( 'NONE',  ( -33.48481952675158624, 76.25000000000001421, -2.578432583507804132 ) ) ;
#7248=CARTESIAN_POINT ( 'NONE',  ( -29.99999999999999645, 4.999999999999999112, -0.9468725184748323365 ) ) ;
#7257=CARTESIAN_POINT ( 'NONE',  ( -15.99999999999998934, 9.999999999999994671, 17.50000000000000000 ) ) ;
#7267=CARTESIAN_POINT ( 'NONE',  ( -15.99999999999999289, 80.00000000000000000, 0.000000000000000000 ) ) ;
#7274=CARTESIAN_POINT ( 'NONE',  ( -16.97782023378069383, 50.47616464312733342, -16.24942753911562932 ) ) ;
#7295=ADVANCED_FACE ( 'NONE', ( #10375 ), #16526, .F. ) ;
#7304=CARTESIAN_POINT ( 'NONE',  ( -28.09482755115952912, 75.66345017797092964, 3.167069675338890722 ) ) ;
#7307=CARTESIAN_POINT ( 'NONE',  ( -27.87934135416876913, 73.83089348061925250, 3.891407385552697384 ) ) ;
#7311=ORIENTED_EDGE ( 'NONE', *, *, #919, .T. ) ;
#7312=AXIS2_PLACEMENT_3D ( 'NONE', #11242, #16122, #19188 ) ;
#7314=ADVANCED_FACE ( 'NONE', ( #12519 ), #16871, .F. ) ;
#7321=VERTEX_POINT ( 'NONE', #1382 ) ;
#7327=EDGE_CURVE ( 'NONE', #681, #8656, #16832, .T. ) ;
#7328=B_SPLINE_CURVE_WITH_KNOTS ( 'NONE', 3,
 ( #4479, #876, #17410, #5626 ),
 .UNSPECIFIED., .F., .F.,
 ( 4, 4 ),
 ( 0.001660622604225808112, 0.002660042459396035584 ),
 .UNSPECIFIED. ) ;
#7332=CARTESIAN_POINT ( 'NONE',  ( -11.09376927746295038, 15.76828681233661378, 0.9644763388355668265 ) ) ;
#7335=EDGE_CURVE ( 'NONE', #491, #3383, #20878, .T. ) ;
#7336=LINE ( 'NONE', #1105, #693 ) ;
#7342=ORIENTED_EDGE ( 'NONE', *, *, #6654, .T. ) ;
#7345=CARTESIAN_POINT ( 'NONE',  ( -23.35826929781130801, 79.96309310684573290, -11.40240185268723394 ) ) ;
#7348=ORIENTED_EDGE ( 'NONE', *, *, #8161, .T. ) ;
#7349=CIRCLE ( 'NONE', #9049, 4.999999999999993783 ) ;
#7360=ORIENTED_EDGE ( 'NONE', *, *, #12072, .T. ) ;
#7371=CARTESIAN_POINT ( 'NONE',  ( -35.00000000000000000, 65.74999999999997158, 1.479896280015810639 ) ) ;
#7376=CARTESIAN_POINT ( 'NONE',  ( -14.51899950647152515, 49.50754942154606653, -12.41803798875660014 ) ) ;
#7383=ORIENTED_EDGE ( 'NONE', *, *, #6654, .F. ) ;
#7389=ORIENTED_EDGE ( 'NONE', *, *, #14339, .T. ) ;
#7391=CARTESIAN_POINT ( 'NONE',  ( -12.88155099176341878, 50.42675226781113196, -16.05345949917837345 ) ) ;
#7392=DIRECTION ( 'NONE',  ( 1.000000000000000000, -0.000000000000000000, -0.000000000000000000 ) ) ;
#7397=CARTESIAN_POINT ( 'NONE',  ( -20.31374355284814825, 64.25000000000000000, -2.528164662410438357 ) ) ;
#7401=DIRECTION ( 'NONE',  ( 0.000000000000000000, 0.000000000000000000, -1.000000000000000000 ) ) ;
#7407=ORIENTED_EDGE ( 'NONE', *, *, #20343, .T. ) ;
#7410=CYLINDRICAL_SURFACE ( 'NONE', #15666, 12.50000000000000000 ) ;
#7413=ORIENTED_EDGE ( 'NONE', *, *, #15108, .T. ) ;
#7416=ORIENTED_EDGE ( 'NONE', *, *, #11156, .T. ) ;
#7437=CARTESIAN_POINT ( 'NONE',  ( -3.510843195177425713, 80.00000000000000000, 0.5205403966592460074 ) ) ;
#7451=CARTESIAN_POINT ( 'NONE',  ( -34.33329038210762718, 64.25000000000000000, -2.193932927905879904 ) ) ;
#7467=FACE_OUTER_BOUND ( 'NONE', #1833, .T. ) ;
#7472=DIRECTION ( 'NONE',  ( 0.000000000000000000, 0.000000000000000000, -1.000000000000000000 ) ) ;
#7476=ORIENTED_EDGE ( 'NONE', *, *, #7335, .T. ) ;
#7482=ADVANCED_FACE ( 'NONE', ( #6750 ), #9730, .F. ) ;
#7489=AXIS2_PLACEMENT_3D ( 'NONE', #9245, #18807, #2702 ) ;
#7490=CARTESIAN_POINT ( 'NONE',  ( -12.17658180577358173, 50.40238676466552192, -15.95319627043026856 ) ) ;
#7505=CARTESIAN_POINT ( 'NONE',  ( -31.93034077464222165, 50.51989448544605921, -8.569845794639380898 ) ) ;
#7506=CARTESIAN_POINT ( 'NONE',  ( -34.66662763442661799, 65.74999999999997158, -1.859747928060476729 ) ) ;
#7516=CARTESIAN_POINT ( 'NONE',  ( -15.67065502568128288, 20.09941697557067997, 12.49999999999999822 ) ) ;
#7522=CARTESIAN_POINT ( 'NONE',  ( -29.99999999999999645, 5.000000000000000000, -15.00000000000000000 ) ) ;
#7528=ORIENTED_EDGE ( 'NONE', *, *, #10029, .T. ) ;
#7530=CARTESIAN_POINT ( 'NONE',  ( 1.312845613648171650, 74.81579058300722807, -1.112382790403132926 ) ) ;
#7532=B_SPLINE_CURVE_WITH_KNOTS ( 'NONE', 3,
 ( #5713, #20250, #10166, #3712, #8596, #13698, #13902, #5510, #20147, #2565, #12099, #2459, #8808, #3825 ),
 .UNSPECIFIED., .F., .F.,
 ( 4, 2, 2, 2, 2, 2, 4 ),
 ( 0.000000000000000000, 0.001404842194932280066, 0.002107263292398419557, 0.002809684389864558832, 0.003512105487330698540, 0.004214526584796837380, 0.005619368779729116796 ),
 .UNSPECIFIED. ) ;
#7542=LINE ( 'NONE', #5730, #5140 ) ;
#7543=DIRECTION ( 'NONE',  ( -1.000000000000000000, -0.000000000000000000, -0.000000000000000000 ) ) ;
#7563=CARTESIAN_POINT ( 'NONE',  ( -35.00000000000000000, 65.74999999999997158, 1.479896280015810639 ) ) ;
#7575=DIRECTION ( 'NONE',  ( 0.000000000000000000, 0.000000000000000000, 1.000000000000000000 ) ) ;
#7594=CARTESIAN_POINT ( 'NONE',  ( -29.99999999999999645, 5.000000000000000000, -10.50000000000000178 ) ) ;
#7595=CARTESIAN_POINT ( 'NONE',  ( -24.72758442336008855, 44.98735168799644413, -8.975511724720679041 ) ) ;
#7597=B_SPLINE_CURVE_WITH_KNOTS ( 'NONE', 3,
 ( #12759, #7968, #20797, #20895, #15841, #17424 ),
 .UNSPECIFIED., .F., .F.,
 ( 4, 2, 4 ),
 ( 0.001660622604225808112, 0.002656748863554461021, 0.003652875122883114146 ),
 .UNSPECIFIED. ) ;
#7600=CARTESIAN_POINT ( 'NONE',  ( -28.07131995261575241, 46.63343660265383051, -3.263164565673607243 ) ) ;
#7611=CARTESIAN_POINT ( 'NONE',  ( 30.10683012259193703, -24.14213562373095456, 4.999999999999997335 ) ) ;
#7613=CARTESIAN_POINT ( 'NONE',  ( -33.12309443379005813, 51.54550291367893067, -5.857582128031854296 ) ) ;
#7614=CARTESIAN_POINT ( 'NONE',  ( -27.65265446014365125, 9.445465779080201685, 4.571190765816516510 ) ) ;
#7625=CARTESIAN_POINT ( 'NONE',  ( -15.99999999999999289, -10.00000000000000000, 5.999999999999989342 ) ) ;
#7636=ORIENTED_EDGE ( 'NONE', *, *, #18062, .F. ) ;
#7637=CARTESIAN_POINT ( 'NONE',  ( -3.376929201035541617, 76.35052269458219598, -2.692414605357459134 ) ) ;
#7639=CARTESIAN_POINT ( 'NONE',  ( -15.99999999999999289, 10.09941697557069418, 4.999999999999989342 ) ) ;
#7643=FACE_OUTER_BOUND ( 'NONE', #12492, .T. ) ;
#7663=CARTESIAN_POINT ( 'NONE',  ( -11.66624079247173995, 12.58454993689042034, 11.72627446870071388 ) ) ;
#7676=AXIS2_PLACEMENT_3D ( 'NONE', #14125, #14333, #9627 ) ;
#7680=EDGE_CURVE ( 'NONE', #13711, #17780, #5493, .T. ) ;
#7683=EDGE_LOOP ( 'NONE', ( #20076, #1556, #10256, #19255 ) ) ;
#7697=CARTESIAN_POINT ( 'NONE',  ( -6.200167922753938576, 50.40944506478484044, -7.783125444142615201 ) ) ;
#7710=CARTESIAN_POINT ( 'NONE',  ( -2.573654215855741612, 77.12664207850482967, -3.593879484356239828 ) ) ;
#7712=EDGE_LOOP ( 'NONE', ( #20486, #14300 ) ) ;
#7715=CARTESIAN_POINT ( 'NONE',  ( 1.402599256620770118, 52.27665093585768830, -4.545845583688177705 ) ) ;
#7716=FACE_OUTER_BOUND ( 'NONE', #2254, .T. ) ;
#7721=CARTESIAN_POINT ( 'NONE',  ( 1.484819526751601559, 76.25000000000000000, -2.578432583507792142 ) ) ;
#7729=CARTESIAN_POINT ( 'NONE',  ( -20.99191269157562090, 15.42836575585571879, 11.45997927866226185 ) ) ;
#7730=CARTESIAN_POINT ( 'NONE',  ( -28.80487160773575184, 69.93605911897407168, 1.714708221108182551 ) ) ;
#7740=CARTESIAN_POINT ( 'NONE',  ( 0.6310778956523167560, 71.62317011047247206, 0.9609777548054254659 ) ) ;
#7751=CARTESIAN_POINT ( 'NONE',  ( -46.99999999999998579, 64.25000000000000000, -2.528164662410438357 ) ) ;
#7755=DIRECTION ( 'NONE',  ( 1.000000000000000000, 0.000000000000000000, 0.000000000000000000 ) ) ;
#7756=ORIENTED_EDGE ( 'NONE', *, *, #8614, .T. ) ;
#7758=CARTESIAN_POINT ( 'NONE',  ( -4.115175346691388292, 73.88542888634934513, 3.878668165723258010 ) ) ;
#7760=CARTESIAN_POINT ( 'NONE',  ( -28.99999999999999289, 0.000000000000000000, 15.00000000000000178 ) ) ;
#7780=CARTESIAN_POINT ( 'NONE',  ( -14.99999999999999645, 0.000000000000000000, 15.00000000000000000 ) ) ;
#7788=CARTESIAN_POINT ( 'NONE',  ( -15.99999999999999289, 0.000000000000000000, 0.000000000000000000 ) ) ;
#7801=CARTESIAN_POINT ( 'NONE',  ( -3.775565802572502960, 47.04367182761800592, -2.628322306727621349 ) ) ;
#7818=CARTESIAN_POINT ( 'NONE',  ( -19.14637054419212348, 50.42580415542552430, -16.04958827719470094 ) ) ;
#7823=CARTESIAN_POINT ( 'NONE',  ( 0.9890147436984468854, 73.25359183295171306, 0.03495786392107397972 ) ) ;
#7831=CARTESIAN_POINT ( 'NONE',  ( -31.85409535283075044, 63.41252023259978898, 2.433313739304557188 ) ) ;
#7840=VERTEX_POINT ( 'NONE', #7905 ) ;
#7841=CARTESIAN_POINT ( 'NONE',  ( -4.425686930326540924, 71.02946758568734253, 4.727326826883592403 ) ) ;
#7842=VECTOR ( 'NONE', #11783, 1000.000000000000000 ) ;
#7852=DIRECTION ( 'NONE',  ( 0.000000000000000000, 0.000000000000000000, -1.000000000000000000 ) ) ;
#7868=CARTESIAN_POINT ( 'NONE',  ( 45.00000000000000000, 5.000000000000000000, 15.00000000000000000 ) ) ;
#7869=CARTESIAN_POINT ( 'NONE',  ( -33.20451348466885833, 77.44204738084620487, -4.113378397039106460 ) ) ;
#7878=CARTESIAN_POINT ( 'NONE',  ( -29.22340388804807532, 78.20541348178687713, -5.222231676846088355 ) ) ;
#7880=CARTESIAN_POINT ( 'NONE',  ( -11.68625644715183931, 65.74999999999995737, -2.528164662410434804 ) ) ;
#7881=ORIENTED_EDGE ( 'NONE', *, *, #13, .F. ) ;
#7883=PLANE ( 'NONE',  #4316 ) ;
#7886=DIRECTION ( 'NONE',  ( 0.000000000000000000, 0.000000000000000000, -1.000000000000000000 ) ) ;
#7895=LINE ( 'NONE', #14397, #5604 ) ;
#7903=CARTESIAN_POINT ( 'NONE',  ( -6.518053481867566390, 50.25229571315650645, -8.166628857475616954 ) ) ;
#7905=CARTESIAN_POINT ( 'NONE',  ( -15.99999999999999289, 9.999999999999994671, -12.50000000000000000 ) ) ;
#7910=CARTESIAN_POINT ( 'NONE',  ( -35.00000000000000000, 65.00000000000000000, -12.50000000000000000 ) ) ;
#7912=CARTESIAN_POINT ( 'NONE',  ( -4.591091843082831581, 79.34446119966882804, -7.911977669603137642 ) ) ;
#7919=CARTESIAN_POINT ( 'NONE',  ( -32.95070415583882806, 56.92051799503307308, 0.1616960027641645703 ) ) ;
#7920=CARTESIAN_POINT ( 'NONE',  ( -28.22159099458506404, 8.920131004072807457, -2.707279339256349004 ) ) ;
#7928=CARTESIAN_POINT ( 'NONE',  ( -27.49344780102824259, 60.03966354978251019, 4.915051137978660556 ) ) ;
#7931=CARTESIAN_POINT ( 'NONE',  ( -14.99999999999999645, -9.999999999999998224, -15.00000000000000000 ) ) ;
#7934=ORIENTED_EDGE ( 'NONE', *, *, #3688, .F. ) ;
#7935=B_SPLINE_CURVE_WITH_KNOTS ( 'NONE', 3,
 ( #20442, #7506, #14215, #10680 ),
 .UNSPECIFIED., .F., .F.,
 ( 4, 4 ),
 ( 8.673617379884035472E-19, 0.001416029653784999084 ),
 .UNSPECIFIED. ) ;
#7939=EDGE_CURVE ( 'NONE', #19075, #3563, #15919, .T. ) ;
#7941=CARTESIAN_POINT ( 'NONE',  ( -2.659465448949789756, 64.25000000000001421, 3.134647201270585271 ) ) ;
#7968=CARTESIAN_POINT ( 'NONE',  ( -20.90620796478638610, 15.76932605263708886, 0.9645878285891481552 ) ) ;
#7970=ORIENTED_EDGE ( 'NONE', *, *, #2675, .T. ) ;
#7971=ORIENTED_EDGE ( 'NONE', *, *, #3416, .T. ) ;
#7972=AXIS2_PLACEMENT_3D ( 'NONE', #9585, #19353, #9892 ) ;
#7977=ORIENTED_EDGE ( 'NONE', *, *, #13910, .F. ) ;
#7988=LINE ( 'NONE', #3333, #1383 ) ;
#7997=DIRECTION ( 'NONE',  ( 1.000000000000000000, -0.000000000000000000, -0.000000000000000000 ) ) ;
#7998=CARTESIAN_POINT ( 'NONE',  ( -25.99999999999999645, 9.999999999999994671, -7.499999999999998224 ) ) ;
#7999=ORIENTED_EDGE ( 'NONE', *, *, #8178, .F. ) ;
#8001=DIRECTION ( 'NONE',  ( 0.000000000000000000, 0.000000000000000000, -1.000000000000000000 ) ) ;
#8003=CARTESIAN_POINT ( 'NONE',  ( -12.36055546714704612, 49.51133710352112871, -11.98200832479694000 ) ) ;
#8008=VERTEX_POINT ( 'NONE', #8322 ) ;
#8009=CARTESIAN_POINT ( 'NONE',  ( -34.00000000000000711, 65.00000000000000000, -27.49999999999999645 ) ) ;
#8010=CARTESIAN_POINT ( 'NONE',  ( -35.00000000000000000, 65.00000000000000000, -12.50000000000000000 ) ) ;
#8011=CARTESIAN_POINT ( 'NONE',  ( 0.6071296115912496738, 78.11617769706943193, -5.220046598459772369 ) ) ;
#8012=ORIENTED_EDGE ( 'NONE', *, *, #17437, .T. ) ;
#8023=CIRCLE ( 'NONE', #17878, 5.999999999999998224 ) ;
#8026=CARTESIAN_POINT ( 'NONE',  ( -28.92176035443840121, 57.78353514853240824, 0.6664698202380902048 ) ) ;
#8027=DIRECTION ( 'NONE',  ( -0.000000000000000000, 1.000000000000000000, -0.000000000000000000 ) ) ;
#8060=CARTESIAN_POINT ( 'NONE',  ( 0.000000000000000000, -10.00000000000000000, 30.00000000000000000 ) ) ;
#8063=CARTESIAN_POINT ( 'NONE',  ( -28.80276981525291546, 76.40330993045616026, -2.758159894511351684 ) ) ;
#8065=EDGE_LOOP ( 'NONE', ( #15250, #396, #15260, #13491, #13467, #7134, #7413 ) ) ;
#8068=ORIENTED_EDGE ( 'NONE', *, *, #14753, .F. ) ;
#8072=VERTEX_POINT ( 'NONE', #10110 ) ;
#8074=CARTESIAN_POINT ( 'NONE',  ( -29.10076314032669842, 78.36047030499236143, -5.510874449650665419 ) ) ;
#8089=DIRECTION ( 'NONE',  ( 0.000000000000000000, -1.000000000000000000, 0.000000000000000000 ) ) ;
#8093=CARTESIAN_POINT ( 'NONE',  ( -29.99999999999999645, 5.000000000000000888, -10.49999999999999822 ) ) ;
#8095=EDGE_LOOP ( 'NONE', ( #15481, #15174, #19355, #11868 ) ) ;
#8102=CARTESIAN_POINT ( 'NONE',  ( -11.35743612562215787, 49.52957768806496119, -11.61502336121733769 ) ) ;
#8113=CARTESIAN_POINT ( 'NONE',  ( -3.576301558931711533, 79.61691370731651318, -9.098688494705450935 ) ) ;
#8123=CARTESIAN_POINT ( 'NONE',  ( -15.28780296042668141, 58.44014375569393849, -4.952210724505383688 ) ) ;
#8134=CARTESIAN_POINT ( 'NONE',  ( -28.93295407825220522, 57.46062458779012161, 0.4842793815437907989 ) ) ;
#8135=CARTESIAN_POINT ( 'NONE',  ( -20.99999999999998224, 15.09941697557068530, 11.45643923738960446 ) ) ;
#8142=ORIENTED_EDGE ( 'NONE', *, *, #7939, .T. ) ;
#8143=CARTESIAN_POINT ( 'NONE',  ( -3.344164530110952605, 66.09831342192623538, 2.470462955493161417 ) ) ;
#8161=EDGE_CURVE ( 'NONE', #4687, #13750, #14578, .T. ) ;
#8162=AXIS2_PLACEMENT_3D ( 'NONE', #14293, #19146, #11085 ) ;
#8165=ORIENTED_EDGE ( 'NONE', *, *, #19118, .T. ) ;
#8168=CIRCLE ( 'NONE', #5453, 4.999999999999989342 ) ;
#8170=LINE ( 'NONE', #8060, #16284 ) ;
#8173=CARTESIAN_POINT ( 'NONE',  ( -14.28172431065628523, 71.25647787916724951, -4.698501153746495795 ) ) ;
#8177=ORIENTED_EDGE ( 'NONE', *, *, #3839, .T. ) ;
#8178=EDGE_CURVE ( 'NONE', #17780, #9666, #8953, .T. ) ;
#8179=CARTESIAN_POINT ( 'NONE',  ( 28.00000000000001066, 65.00000000000000000, -12.50000000000000000 ) ) ;
#8181=CARTESIAN_POINT ( 'NONE',  ( -31.83924231307694441, 66.25779166050591584, 2.455816886943472888 ) ) ;
#8203=FACE_OUTER_BOUND ( 'NONE', #10281, .T. ) ;
#8208=CARTESIAN_POINT ( 'NONE',  ( -10.07778552363583380, 45.21291330008718745, -11.01476690536905956 ) ) ;
#8212=CARTESIAN_POINT ( 'NONE',  ( -4.250339552839886181, 57.32441097052598877, 4.267670548753550008 ) ) ;
#8214=EDGE_CURVE ( 'NONE', #10554, #7321, #17342, .T. ) ;
#8219=VERTEX_POINT ( 'NONE', #18724 ) ;
#8225=CARTESIAN_POINT ( 'NONE',  ( -19.29903332301958585, 60.14018031781252205, -3.758841495318848480 ) ) ;
#8234=EDGE_CURVE ( 'NONE', #7840, #2330, #11867, .T. ) ;
#8237=CARTESIAN_POINT ( 'NONE',  ( -28.84012200976501461, 59.46807757785196458, 1.471601637521282591 ) ) ;
#8253=ORIENTED_EDGE ( 'NONE', *, *, #919, .F. ) ;
#8277=UNCERTAINTY_MEASURE_WITH_UNIT (LENGTH_MEASURE( 1.000000000000000082E-05 ), #15806, 'distance_accuracy_value', 'NONE');
#8282=CARTESIAN_POINT ( 'NONE',  ( -32.60712961159122614, 78.11617769706940351, -5.220046598459701315 ) ) ;
#8286=AXIS2_PLACEMENT_3D ( 'NONE', #1814, #2233, #5389 ) ;
#8307=CARTESIAN_POINT ( 'NONE',  ( -30.00000000000002842, 4.999999999999995559, -8.933394465404589369 ) ) ;
#8313=CARTESIAN_POINT ( 'NONE',  ( -3.625355398317132494, 51.79533773540889285, 1.819264427481864121 ) ) ;
#8319=CARTESIAN_POINT ( 'NONE',  ( -3.548890045384964331, 48.22447992834113251, -1.142799159744782411 ) ) ;
#8321=VECTOR ( 'NONE', #3682, 1000.000000000000000 ) ;
#8322=CARTESIAN_POINT ( 'NONE',  ( -15.99999999999999289, 20.09941697557067997, 4.999999999999989342 ) ) ;
#8327=ORIENTED_EDGE ( 'NONE', *, *, #19951, .T. ) ;
#8329=DIRECTION ( 'NONE',  ( 0.000000000000000000, 0.000000000000000000, -1.000000000000000000 ) ) ;
#8332=ADVANCED_FACE ( 'NONE', ( #7467 ), #18824, .F. ) ;
#8333=CARTESIAN_POINT ( 'NONE',  ( -16.71639762958279007, 58.44083456968236590, -4.951609446663259639 ) ) ;
#8337=CARTESIAN_POINT ( 'NONE',  ( -14.27770786790704705, 58.73247755281146709, -4.704935945893314653 ) ) ;
#8345=EDGE_CURVE ( 'NONE', #3730, #4124, #7988, .T. ) ;
#8347=CARTESIAN_POINT ( 'NONE',  ( -28.16085501120128853, 46.85610706404197146, -2.909190404198925162 ) ) ;
#8357=ORIENTED_EDGE ( 'NONE', *, *, #19788, .T. ) ;
#8375=CARTESIAN_POINT ( 'NONE',  ( -14.99999999999999822, 0.000000000000000000, -28.99999999999999645 ) ) ;
#8385=VECTOR ( 'NONE', #20340, 1000.000000000000000 ) ;
#8392=CARTESIAN_POINT ( 'NONE',  ( -23.11077747421012063, 79.96752057144479409, -11.48167302094428344 ) ) ;
#8402=CYLINDRICAL_SURFACE ( 'NONE', #10480, 13.99999999999999822 ) ;
#8403=DIRECTION ( 'NONE',  ( 0.000000000000000000, 0.000000000000000000, -1.000000000000000000 ) ) ;
#8405=DIRECTION ( 'NONE',  ( 0.000000000000000000, 0.000000000000000000, -1.000000000000000000 ) ) ;
#8413=CARTESIAN_POINT ( 'NONE',  ( -26.22872419829098334, 5.421422414486862351, -7.194700298646708347 ) ) ;
#8417=CARTESIAN_POINT ( 'NONE',  ( -8.151266174553969179, 45.02035806555345943, -9.759823581491495759 ) ) ;
#8421=CARTESIAN_POINT ( 'NONE',  ( -3.954476518211411662, 54.76190936792474417, 3.362518328805365719 ) ) ;
#8425=EDGE_CURVE ( 'NONE', #7321, #4222, #2390, .T. ) ;
#8430=ORIENTED_EDGE ( 'NONE', *, *, #6429, .T. ) ;
#8431=DIRECTION ( 'NONE',  ( 1.000000000000000000, 0.000000000000000000, 0.000000000000000000 ) ) ;
#8433=ORIENTED_EDGE ( 'NONE', *, *, #12719, .F. ) ;
#8434=ORIENTED_EDGE ( 'NONE', *, *, #18496, .T. ) ;
#8440=DIRECTION ( 'NONE',  ( 0.000000000000000000, -1.000000000000000000, 0.000000000000000000 ) ) ;
#8449=CARTESIAN_POINT ( 'NONE',  ( -28.47807888696556589, 50.32121178641160242, 0.7806563195649840470 ) ) ;
#8457=AXIS2_PLACEMENT_3D ( 'NONE', #4514, #20502, #7886 ) ;
#8461=DIRECTION ( 'NONE',  ( 0.000000000000000000, 0.000000000000000000, -1.000000000000000000 ) ) ;
#8488=CARTESIAN_POINT ( 'NONE',  ( -12.98588573640857291, 70.25594724513304357, -3.991311237440293258 ) ) ;
#8492=EDGE_CURVE ( 'NONE', #15613, #17576, #1370, .T. ) ;
#8501=CARTESIAN_POINT ( 'NONE',  ( -15.99999999999999289, 79.99999999999998579, -12.50000000000000178 ) ) ;
#8506=CIRCLE ( 'NONE', #7489, 4.999999999999990230 ) ;
#8509=LINE ( 'NONE', #1949, #14989 ) ;
#8514=VERTEX_POINT ( 'NONE', #15221 ) ;
#8519=CARTESIAN_POINT ( 'NONE',  ( -7.416086753897887185, 79.99999999992817834, -9.098350519373953560 ) ) ;
#8529=CARTESIAN_POINT ( 'NONE',  ( -27.42820750412292341, 6.346396126445347008, 5.151021229765904152 ) ) ;
#8532=EDGE_LOOP ( 'NONE', ( #16918, #13121, #18521, #20889, #8165, #6117, #5147, #18912 ) ) ;
#8534=CARTESIAN_POINT ( 'NONE',  ( -5.556399631426875985, 45.18150654375704534, -6.911722607583233646 ) ) ;
#8537=CARTESIAN_POINT ( 'NONE',  ( -3.526256370528186412, 48.49133988427076503, -0.8569032390966567769 ) ) ;
#8538=CARTESIAN_POINT ( 'NONE',  ( -2.443633760204237504, 79.40511245435270382, -8.308716123878882698 ) ) ;
#8547=VERTEX_POINT ( 'NONE', #2060 ) ;
#8561=DIRECTION ( 'NONE',  ( 0.000000000000000000, 1.000000000000000000, 0.000000000000000000 ) ) ;
#8562=DIRECTION ( 'NONE',  ( -0.000000000000000000, -1.000000000000000000, -0.000000000000000000 ) ) ;
#8563=CARTESIAN_POINT ( 'NONE',  ( -33.41199867414998437, 54.49694147696414603, -1.784705491317941206 ) ) ;
#8596=CARTESIAN_POINT ( 'NONE',  ( -2.018562491348669496, 65.74999999999998579, 2.826871295670243978 ) ) ;
#8597=CARTESIAN_POINT ( 'NONE',  ( -15.28360237041720282, 71.55916543031763410, -4.951609446663259639 ) ) ;
#8612=CARTESIAN_POINT ( 'NONE',  ( 30.00000000000000000, -9.999999999999998224, 15.00000000000000000 ) ) ;
#8614=EDGE_CURVE ( 'NONE', #20919, #1328, #19955, .T. ) ;
#8616=CARTESIAN_POINT ( 'NONE',  ( -31.34819869032959261, 64.25000000000002842, 2.481238266578627893 ) ) ;
#8620=CARTESIAN_POINT ( 'NONE',  ( 28.00000000000001066, 65.00000000000000000, -12.50000000000000000 ) ) ;
#8621=CARTESIAN_POINT ( 'NONE',  ( -4.530168698509680070, 79.99999999986593480, -4.984538917061887453 ) ) ;
#8626=EDGE_CURVE ( 'NONE', #166, #4564, #11920, .T. ) ;
#8627=CARTESIAN_POINT ( 'NONE',  ( -14.99999999999999822, -10.00000000000000000, -28.99999999999999645 ) ) ;
#8631=AXIS2_PLACEMENT_3D ( 'NONE', #8818, #10822, #17199 ) ;
#8632=CARTESIAN_POINT ( 'NONE',  ( -26.39566432206697755, 9.975777012415697698, 6.949400359526464399 ) ) ;
#8634=EDGE_CURVE ( 'NONE', #4202, #19075, #7336, .T. ) ;
#8640=CARTESIAN_POINT ( 'NONE',  ( -3.276752736765743634, 61.69737001983726543, 2.155802286817233959 ) ) ;
#8641=CARTESIAN_POINT ( 'NONE',  ( 1.486836232935293767, 76.55853692374149944, -2.936780385859808717 ) ) ;
#8646=AXIS2_PLACEMENT_3D ( 'NONE', #18032, #15297, #7401 ) ;
#8654=B_SPLINE_CURVE_WITH_KNOTS ( 'NONE', 3,
 ( #1627, #8181, #143, #16162, #14579, #40, #6479, #11478, #3116, #17853, #19426, #14687, #11066, #6582 ),
 .UNSPECIFIED., .F., .F.,
 ( 4, 2, 2, 2, 2, 2, 4 ),
 ( 0.000000000000000000, 0.001520696258467074333, 0.003041392516934148665, 0.006082785033868297331, 0.007603481292335390745, 0.009124177550802484160, 0.01216557006773670568 ),
 .UNSPECIFIED. ) ;
#8656=VERTEX_POINT ( 'NONE', #19119 ) ;
#8661=VERTEX_POINT ( 'NONE', #20272 ) ;
#8663=CARTESIAN_POINT ( 'NONE',  ( -19.99144900083270215, 68.18358604705119319, -3.013858250467852606 ) ) ;
#8670=CARTESIAN_POINT ( 'NONE',  ( -28.62507391571850945, 53.64368112681762568, -2.695303598069996642 ) ) ;
#8684=DIRECTION ( 'NONE',  ( 0.000000000000000000, 0.000000000000000000, -1.000000000000000000 ) ) ;
#8690=AXIS2_PLACEMENT_3D ( 'NONE', #19494, #532, #11665 ) ;
#8691=DIRECTION ( 'NONE',  ( 0.03124427847888232648, 0.6611148994991496997, -0.7496338337632335591 ) ) ;
#8693=CARTESIAN_POINT ( 'NONE',  ( 30.10683012259193703, 0.000000000000000000, -5.999999999999998224 ) ) ;
#8695=CARTESIAN_POINT ( 'NONE',  ( -33.31284561364699215, 74.81579058300519591, -1.112382790401626798 ) ) ;
#8698=ORIENTED_EDGE ( 'NONE', *, *, #4826, .T. ) ;
#8709=ORIENTED_EDGE ( 'NONE', *, *, #19087, .T. ) ;
#8725=DIRECTION ( 'NONE',  ( 1.000000000000000000, 0.000000000000000000, 0.000000000000000000 ) ) ;
#8733=CARTESIAN_POINT ( 'NONE',  ( -33.49470602546865905, 76.40689540430931004, -2.756335249929798614 ) ) ;
#8748=CARTESIAN_POINT ( 'NONE',  ( 30.00000000000000355, 5.000000000000000000, -15.00000000000000000 ) ) ;
#8751=ORIENTED_EDGE ( 'NONE', *, *, #3208, .F. ) ;
#8756=EDGE_CURVE ( 'NONE', #1288, #8514, #20232, .T. ) ;
#8764=ORIENTED_EDGE ( 'NONE', *, *, #7026, .T. ) ;
#8766=CARTESIAN_POINT ( 'NONE',  ( -20.13425257954909142, 67.51366979390380152, -2.814775708409672728 ) ) ;
#8774=CARTESIAN_POINT ( 'NONE',  ( -28.77462657304674565, 54.25663578079195304, -2.022313059153934223 ) ) ;
#8777=EDGE_CURVE ( 'NONE', #17576, #15613, #6110, .T. ) ;
#8786=DIRECTION ( 'NONE',  ( 0.000000000000000000, -1.000000000000000000, 0.000000000000000000 ) ) ;
#8789=EDGE_LOOP ( 'NONE', ( #13994, #9032, #15031, #8433, #11341 ) ) ;
#8792=EDGE_CURVE ( 'NONE', #20070, #3073, #8170, .T. ) ;
#8801=CIRCLE ( 'NONE', #6077, 5.000000000000000888 ) ;
#8803=CARTESIAN_POINT ( 'NONE',  ( -28.36631829605002508, 78.08772077735660844, 1.916778294987758313 ) ) ;
#8808=CARTESIAN_POINT ( 'NONE',  ( -4.498192030073390413, 65.74999999999998579, 4.917728941844615953 ) ) ;
#8812=DIRECTION ( 'NONE',  ( 1.000000000000000000, 1.110223024625156540E-15, 0.000000000000000000 ) ) ;
#8815=EDGE_LOOP ( 'NONE', ( #12323, #16357 ) ) ;
#8817=CARTESIAN_POINT ( 'NONE',  ( -24.06039977493734483, 79.94564677075823056, -11.17290160265476828 ) ) ;
#8818=CARTESIAN_POINT ( 'NONE',  ( -14.99999999999999645, -10.00000000000000000, -15.00000000000000000 ) ) ;
#8827=CIRCLE ( 'NONE', #5421, 4.999999999999989342 ) ;
#8829=DIRECTION ( 'NONE',  ( 0.000000000000000000, -1.000000000000000000, 0.000000000000000000 ) ) ;
#8830=AXIS2_PLACEMENT_3D ( 'NONE', #1257, #2850, #1463 ) ;
#8832=DIRECTION ( 'NONE',  ( -0.000000000000000000, 1.000000000000000000, -0.000000000000000000 ) ) ;
#8836=CARTESIAN_POINT ( 'NONE',  ( -28.99999999999999289, -10.00000000000000000, 15.00000000000000178 ) ) ;
#8837=LINE ( 'NONE', #1318, #14656 ) ;
#8840=AXIS2_PLACEMENT_3D ( 'NONE', #7788, #19543, #12997 ) ;
#8850=DIRECTION ( 'NONE',  ( 0.000000000000000000, 0.000000000000000000, -1.000000000000000000 ) ) ;
#8858=CARTESIAN_POINT ( 'NONE',  ( 28.00000000000001066, 64.25000000000000000, -1.525597966175989972 ) ) ;
#8860=CARTESIAN_POINT ( 'NONE',  ( -35.00000000000000000, 65.74999999999997158, -1.525597966176003961 ) ) ;
#8861=CIRCLE ( 'NONE', #7164, 5.000000000000001776 ) ;
#8868=CARTESIAN_POINT ( 'NONE',  ( -16.88867936483986654, 71.52687714446561529, -4.923512665565291435 ) ) ;
#8872=DIRECTION ( 'NONE',  ( 0.000000000000000000, -1.000000000000000000, 0.000000000000000000 ) ) ;
#8876=CARTESIAN_POINT ( 'NONE',  ( -29.20450150413485346, 50.01656837298652647, -11.74597530808301649 ) ) ;
#8881=CARTESIAN_POINT ( 'NONE',  ( -28.46516275735407220, 48.23356369194445392, -1.109776825402767120 ) ) ;
#8886=EDGE_LOOP ( 'NONE', ( #15608, #18316, #13262, #7360 ) ) ;
#8888=CARTESIAN_POINT ( 'NONE',  ( -15.99999999999999289, 15.09941697557068530, 0.9999999999999991118 ) ) ;
#8901=EDGE_CURVE ( 'NONE', #1440, #12607, #12216, .T. ) ;
#8917=AXIS2_PLACEMENT_3D ( 'NONE', #639, #6659, #11453 ) ;
#8931=AXIS2_PLACEMENT_3D ( 'NONE', #3917, #18768, #752 ) ;
#8935=CARTESIAN_POINT ( 'NONE',  ( -15.47785846381593089, 80.00000165566777355, -12.49590370130045258 ) ) ;
#8940=CARTESIAN_POINT ( 'NONE',  ( -15.99999999999999289, 0.000000000000000000, 5.999999999999989342 ) ) ;
#8950=CARTESIAN_POINT ( 'NONE',  ( 30.00000000000000000, 5.000000000000000000, 15.00000000000000000 ) ) ;
#8952=CARTESIAN_POINT ( 'NONE',  ( -34.33334827330879335, 64.25000000000000000, 2.147472525011941080 ) ) ;
#8953=LINE ( 'NONE', #18193, #9799 ) ;
#8955=VERTEX_POINT ( 'NONE', #8009 ) ;
#8957=CARTESIAN_POINT ( 'NONE',  ( 0.000000000000000000, 5.000000000000000000, 30.00000000000000000 ) ) ;
#8970=LINE ( 'NONE', #4213, #19603 ) ;
#8973=CARTESIAN_POINT ( 'NONE',  ( -19.73795054555117545, 45.44664558820969802, -11.93297875370773298 ) ) ;
#8978=ADVANCED_FACE ( 'NONE', ( #4639 ), #17371, .T. ) ;
#8986=CARTESIAN_POINT ( 'NONE',  ( 1.154989429455318684, 55.96508055892482503, -0.5199069304187589058 ) ) ;
#8989=EDGE_LOOP ( 'NONE', ( #6216, #14067, #16328, #9498 ) ) ;
#8996=FACE_BOUND ( 'NONE', #7712, .T. ) ;
#8997=CARTESIAN_POINT ( 'NONE',  ( -14.37689184831195632, 19.83987654191486172, 12.39791892878506374 ) ) ;
#8999=DIRECTION ( 'NONE',  ( -8.673617379884032514E-16, -0.7500000000000004441, -0.6614378277661471239 ) ) ;
#9000=DIRECTION ( 'NONE',  ( -0.000000000000000000, -0.000000000000000000, 1.000000000000000000 ) ) ;
#9002=AXIS2_PLACEMENT_3D ( 'NONE', #13631, #16801, #2279 ) ;
#9005=CARTESIAN_POINT ( 'NONE',  ( -32.38807006469330929, 70.47620764902667645, 1.501429235142507590 ) ) ;
#9010=VERTEX_POINT ( 'NONE', #4737 ) ;
#9016=CARTESIAN_POINT ( 'NONE',  ( -14.99999999999999645, 0.000000000000000000, -28.99999999999999645 ) ) ;
#9032=ORIENTED_EDGE ( 'NONE', *, *, #1655, .T. ) ;
#9038=ORIENTED_EDGE ( 'NONE', *, *, #16424, .F. ) ;
#9039=VERTEX_POINT ( 'NONE', #17782 ) ;
#9042=CARTESIAN_POINT ( 'NONE',  ( -14.22556875492139561, 10.42203463021438559, 12.37434949811833818 ) ) ;
#9044=CARTESIAN_POINT ( 'NONE',  ( -25.10457607615188991, 79.90025503832140430, -10.76317361290839436 ) ) ;
#9049=AXIS2_PLACEMENT_3D ( 'NONE', #2608, #17434, #9353 ) ;
#9052=CYLINDRICAL_SURFACE ( 'NONE', #10908, 5.999999999999998224 ) ;
#9053=ORIENTED_EDGE ( 'NONE', *, *, #6924, .T. ) ;
#9058=CARTESIAN_POINT ( 'NONE',  ( -34.00000000000000711, 65.00000000000000000, -12.50000000000000000 ) ) ;
#9064=AXIS2_PLACEMENT_3D ( 'NONE', #12739, #2992, #7852 ) ;
#9066=CARTESIAN_POINT ( 'NONE',  ( -20.99999999999998934, 14.77053021905504693, 11.45643923738960446 ) ) ;
#9067=PRODUCT_DEFINITION_SHAPE ( 'NONE', 'NONE',  #19727 ) ;
#9073=EDGE_CURVE ( 'NONE', #12607, #1135, #13913, .T. ) ;
#9075=CARTESIAN_POINT ( 'NONE',  ( -14.15118760488712013, 49.50739088371899754, -12.36866518513531332 ) ) ;
#9078=( BOUNDED_SURFACE ( )  B_SPLINE_SURFACE ( 3, 2, ( 
 ( #1798, #4755, #17597 ),
 ( #6332, #17494, #3070 ),
 ( #17912, #19477, #7831 ),
 ( #19184, #11237, #17707 ),
 ( #4656, #9520, #1483 ),
 ( #7928, #9624, #4863 ),
 ( #20859, #1687, #17801 ),
 ( #14537, #8237, #201 ),
 ( #16119, #11334, #1585 ),
 ( #12623, #8026, #3272 ),
 ( #9724, #8134, #107 ),
 ( #13038, #16522, #20010 ),
 ( #19691, #5162, #520 ),
 ( #621, #19582, #11652 ),
 ( #18013, #10027, #5264 ),
 ( #2318, #13137, #417 ),
 ( #3483, #8774, #8563 ),
 ( #8449, #9928, #14952 ),
 ( #15062, #8670, #18213 ),
 ( #6863, #13348, #301 ),
 ( #10131, #16422, #5366 ),
 ( #6746, #5474, #13243 ),
 ( #1898, #3678, #3582 ),
 ( #19795, #2001, #11753 ),
 ( #8347, #14851, #18114 ),
 ( #16624, #2113, #6965 ),
 ( #13452, #15270, #5059 ),
 ( #6642, #3895, #19900 ),
 ( #11538, #11858, #18322 ),
 ( #10348, #3791, #10241 ),
 ( #16732, #2212, #15167 ),
 ( #7074, #13558, #18426 ),
 ( #11967, #16835, #18743 ),
 ( #18944, #20426, #4003 ),
 ( #2420, #15685, #8876 ),
 ( #7595, #5577, #14087 ),
 ( #13870, #5791, #5681 ),
 ( #12171, #16937, #1150 ),
 ( #20320, #15575, #10452 ),
 ( #10773, #5891, #20524 ),
 ( #5995, #12488, #20116 ),
 ( #12391, #2528, #4112 ),
 ( #13984, #4216, #18637 ),
 ( #8973, #4422, #13663 ),
 ( #10567, #10882, #9178 ),
 ( #2736, #18846, #4320 ),
 ( #17364, #15375, #17250 ),
 ( #2841, #827, #7180 ),
 ( #9279, #17150, #7274 ),
 ( #2634, #15475, #18534 ),
 ( #12288, #13764, #726 ),
 ( #932, #7376, #10664 ),
 ( #12067, #9075, #20213 ),
 ( #17050, #1038, #7490 ),
 ( #6513, #8003, #1250 ),
 ( #14509, #8102, #20935 ),
 ( #13012, #14616, #16092 ),
 ( #1662, #4729, #11097 ),
 ( #15992, #15879, #17887 ),
 ( #1558, #11409, #19451 ),
 ( #12594, #15782, #17570 ),
 ( #20627, #17773, #78 ),
 ( #3242, #12698, #14303 ),
 ( #9382, #14198, #11308 ),
 ( #1457, #4630, #3349 ),
 ( #4934, #7903, #20738 ),
 ( #9489, #7697, #6206 ),
 ( #9594, #6099, #6408 ),
 ( #9697, #6306, #12906 ),
 ( #19359, #19261, #19057 ),
 ( #3040, #19156, #16192 ),
 ( #4835, #1352, #11203 ),
 ( #4530, #10997, #17465 ),
 ( #20830, #2943, #14402 ),
 ( #7801, #12801, #17678 ),
 ( #3148, #1870, #19664 ),
 ( #5034, #5137, #2188 ),
 ( #8319, #14823, #3654 ),
 ( #8537, #595, #3454 ),
 ( #3553, #7045, #5236 ),
 ( #9903, #11727, #9998 ),
 ( #11625, #13529, #18189 ),
 ( #387, #16492, #18088 ),
 ( #16396, #15038, #13323 ),
 ( #16596, #11510, #273 ),
 ( #6718, #19979, #19556 ),
 ( #13214, #14922, #1973 ),
 ( #8421, #10107, #173 ),
 ( #6839, #16710, #19770 ),
 ( #6617, #2083, #496 ),
 ( #8212, #6935, #5442 ),
 ( #16292, #13426, #17988 ),
 ( #19871, #14719, #11830 ),
 ( #5337, #18290, #3764 ),
 ( #10216, #8640, #13111 ),
 ( #15140, #11941, #18401 ),
 ( #9802, #1768, #17024 ),
 ( #5871, #18608, #10321 ) ),
 .UNSPECIFIED., .F., .F., .T. ) 
 B_SPLINE_SURFACE_WITH_KNOTS ( ( 4, 2, 2, 2, 2, 2, 2, 2, 2, 2, 2, 2, 2, 2, 2, 2, 2, 2, 2, 2, 2, 2, 2, 2, 2, 2, 2, 2, 2, 2, 2, 2, 2, 2, 2, 2, 2, 2, 2, 2, 2, 2, 2, 2, 2, 2, 2, 2, 4 ),
 ( 3, 3 ),
 ( 0.05371843306266368967, 0.05659148630217877840, 0.05802801292193632277, 0.05946453954169386713, 0.06233759278120895586, 0.06377411940096650023, 0.06521064602072404459, 0.06808369926023913332, 0.06952022587999667769, 0.07095675249975422205, 0.07382980573926931078, 0.07526633235902685515, 0.07670285897878439951, 0.07957591221829948824, 0.08101243883805703261, 0.08244896545781457697, 0.08388549207757212134, 0.08532201869732966570, 0.08819507193684475443, 0.08963159855660229880, 0.09106812517635984316, 0.09394117841587493190, 0.09537770503563247626, 0.09681423165539002063, 0.09968728489490510936, 0.1011238115146626537, 0.1025603381344201981, 0.1054333913739352868, 0.1068699179936928312, 0.1083064446134503755, 0.1111794978529654643, 0.1126160244727230086, 0.1140525510924805530, 0.1169256043319956417, 0.1183621309517531861, 0.1197986575715107305, 0.1226717108110258192, 0.1241082374307833636, 0.1255447640505409079, 0.1269812906702984523, 0.1284178172900559967, 0.1312908705295710854, 0.1327273971493286298, 0.1341639237690861741, 0.1370369770086012629, 0.1384735036283588072, 0.1399100302481163516, 0.1427830834876314403, 0.1456561367271465290 ),
 ( 0.000000000000000000, 1.000000000000000000 ),
 .UNSPECIFIED. ) 
 GEOMETRIC_REPRESENTATION_ITEM ( )  RATIONAL_B_SPLINE_SURFACE ( (
 ( 1.000000000000000000, 0.8451295721185223542, 1.000000000000000000),
 ( 1.000000000000000000, 0.8449004303875792266, 1.000000000000000000),
 ( 1.000000000000000000, 0.8430801628613031617, 1.000000000000000000),
 ( 1.000000000000000000, 0.8379707563242198010, 1.000000000000000000),
 ( 1.000000000000000000, 0.8358658383963908367, 1.000000000000000000),
 ( 1.000000000000000000, 0.8309676740331579659, 1.000000000000000000),
 ( 1.000000000000000000, 0.8281679717263343843, 1.000000000000000000),
 ( 1.000000000000000000, 0.8188015739685772232, 1.000000000000000000),
 ( 1.000000000000000000, 0.8112657144558387268, 1.000000000000000000),
 ( 1.000000000000000000, 0.7983672344561800749, 1.000000000000000000),
 ( 1.000000000000000000, 0.7937839858167325957, 1.000000000000000000),
 ( 1.000000000000000000, 0.7842772446598291758, 1.000000000000000000),
 ( 1.000000000000000000, 0.7793499137115288411, 1.000000000000000000),
 ( 1.000000000000000000, 0.7641988213884888248, 1.000000000000000000),
 ( 1.000000000000000000, 0.7535972611492264273, 1.000000000000000000),
 ( 1.000000000000000000, 0.7376610632163976833, 1.000000000000000000),
 ( 1.000000000000000000, 0.7323451700871047576, 1.000000000000000000),
 ( 1.000000000000000000, 0.7218574730905190640, 1.000000000000000000),
 ( 1.000000000000000000, 0.7167041927396170520, 1.000000000000000000),
 ( 1.000000000000000000, 0.7019988979607418855, 1.000000000000000000),
 ( 1.000000000000000000, 0.6931069249354639972, 1.000000000000000000),
 ( 1.000000000000000000, 0.6821959854549815017, 1.000000000000000000),
 ( 1.000000000000000000, 0.6789533902147232292, 1.000000000000000000),
 ( 1.000000000000000000, 0.6735202903929765617, 1.000000000000000000),
 ( 1.000000000000000000, 0.6713489072053013818, 1.000000000000000000),
 ( 1.000000000000000000, 0.6665638323410731925, 1.000000000000000000),
 ( 1.000000000000000000, 0.6656972691007314591, 1.000000000000000000),
 ( 1.000000000000000000, 0.6679527106063430919, 1.000000000000000000),
 ( 1.000000000000000000, 0.6693061893886460556, 1.000000000000000000),
 ( 1.000000000000000000, 0.6730365072794786130, 1.000000000000000000),
 ( 1.000000000000000000, 0.6754117021867901416, 1.000000000000000000),
 ( 1.000000000000000000, 0.6810047018611226077, 1.000000000000000000),
 ( 1.000000000000000000, 0.6842223828699847132, 1.000000000000000000),
 ( 1.000000000000000000, 0.6913184916867489704, 1.000000000000000000),
 ( 1.000000000000000000, 0.6952162037222894275, 1.000000000000000000),
 ( 1.000000000000000000, 0.7074730050970403639, 1.000000000000000000),
 ( 1.000000000000000000, 0.7163322597878015729, 1.000000000000000000),
 ( 1.000000000000000000, 0.7295517996625942025, 1.000000000000000000),
 ( 1.000000000000000000, 0.7339499638009396865, 1.000000000000000000),
 ( 1.000000000000000000, 0.7425745160330512462, 1.000000000000000000),
 ( 1.000000000000000000, 0.7467701689946989463, 1.000000000000000000),
 ( 1.000000000000000000, 0.7587200212276741240, 1.000000000000000000),
 ( 1.000000000000000000, 0.7658780977019831182, 1.000000000000000000),
 ( 1.000000000000000000, 0.7748278484315241910, 1.000000000000000000),
 ( 1.000000000000000000, 0.7775215145640017589, 1.000000000000000000),
 ( 1.000000000000000000, 0.7821966049398736409, 1.000000000000000000),
 ( 1.000000000000000000, 0.7841643293397753123, 1.000000000000000000),
 ( 1.000000000000000000, 0.7889180347041169217, 1.000000000000000000),
 ( 1.000000000000000000, 0.7905538983596147595, 1.000000000000000000),
 ( 1.000000000000000000, 0.7905770084924903518, 1.000000000000000000),
 ( 1.000000000000000000, 0.7901767721866111982, 1.000000000000000000),
 ( 1.000000000000000000, 0.7885605096290441152, 1.000000000000000000),
 ( 1.000000000000000000, 0.7873530734365258299, 1.000000000000000000),
 ( 1.000000000000000000, 0.7826096900989555349, 1.000000000000000000),
 ( 1.000000000000000000, 0.7779500639155249031, 1.000000000000000000),
 ( 1.000000000000000000, 0.7690412136372090091, 1.000000000000000000),
 ( 1.000000000000000000, 0.7657396504301140494, 1.000000000000000000),
 ( 1.000000000000000000, 0.7586220519610614721, 1.000000000000000000),
 ( 1.000000000000000000, 0.7548291205712890362, 1.000000000000000000),
 ( 1.000000000000000000, 0.7429250358377615937, 1.000000000000000000),
 ( 1.000000000000000000, 0.7342788820070000888, 1.000000000000000000),
 ( 1.000000000000000000, 0.7210645840206886259, 1.000000000000000000),
 ( 1.000000000000000000, 0.7166062187610443557, 1.000000000000000000),
 ( 1.000000000000000000, 0.7078513950284187617, 1.000000000000000000),
 ( 1.000000000000000000, 0.7035928640278642510, 1.000000000000000000),
 ( 1.000000000000000000, 0.6914457770771308409, 1.000000000000000000),
 ( 1.000000000000000000, 0.6841809009208725811, 1.000000000000000000),
 ( 1.000000000000000000, 0.6756975108818989995, 1.000000000000000000),
 ( 1.000000000000000000, 0.6732685451421130951, 1.000000000000000000),
 ( 1.000000000000000000, 0.6694443308151706296, 1.000000000000000000),
 ( 1.000000000000000000, 0.6680762773069750526, 1.000000000000000000),
 ( 1.000000000000000000, 0.6657056734595532266, 1.000000000000000000),
 ( 1.000000000000000000, 0.6664547459774202709, 1.000000000000000000),
 ( 1.000000000000000000, 0.6711610830150476215, 1.000000000000000000),
 ( 1.000000000000000000, 0.6733389247384340415, 1.000000000000000000),
 ( 1.000000000000000000, 0.6787002311037058089, 1.000000000000000000),
 ( 1.000000000000000000, 0.6818858631847106722, 1.000000000000000000),
 ( 1.000000000000000000, 0.6891021881274688177, 1.000000000000000000),
 ( 1.000000000000000000, 0.6931327393535783310, 1.000000000000000000),
 ( 1.000000000000000000, 0.7018714184841962078, 1.000000000000000000),
 ( 1.000000000000000000, 0.7066008739865929922, 1.000000000000000000),
 ( 1.000000000000000000, 0.7213821357138887613, 1.000000000000000000),
 ( 1.000000000000000000, 0.7319733230681478853, 1.000000000000000000),
 ( 1.000000000000000000, 0.7479842531354111701, 1.000000000000000000),
 ( 1.000000000000000000, 0.7533449566548310328, 1.000000000000000000),
 ( 1.000000000000000000, 0.7639785367744996725, 1.000000000000000000),
 ( 1.000000000000000000, 0.7692354322323328164, 1.000000000000000000),
 ( 1.000000000000000000, 0.7844906279380156056, 1.000000000000000000),
 ( 1.000000000000000000, 0.7940371516267079599, 1.000000000000000000),
 ( 1.000000000000000000, 0.8069106371822711843, 1.000000000000000000),
 ( 1.000000000000000000, 0.8109620220656993395, 1.000000000000000000),
 ( 1.000000000000000000, 0.8185080840883726117, 1.000000000000000000),
 ( 1.000000000000000000, 0.8220058205555477171, 1.000000000000000000),
 ( 1.000000000000000000, 0.8314117683381576640, 1.000000000000000000),
 ( 1.000000000000000000, 0.8362949755366669846, 1.000000000000000000),
 ( 1.000000000000000000, 0.8430419324072143672, 1.000000000000000000),
 ( 1.000000000000000000, 0.8449066468994074208, 1.000000000000000000),
 ( 1.000000000000000000, 0.8451313959173227808, 1.000000000000000000) ) ) 
 REPRESENTATION_ITEM ( '' )  SURFACE ( )  );
#9087=EDGE_CURVE ( 'NONE', #1135, #15273, #15066, .T. ) ;
#9090=CARTESIAN_POINT ( 'NONE',  ( -25.87449106562930368, 50.06942782642894230, -13.97928078101991289 ) ) ;
#9091=CARTESIAN_POINT ( 'NONE',  ( -28.06278917795930283, 9.095778419061115727, -3.341700078353888159 ) ) ;
#9096=CARTESIAN_POINT ( 'NONE',  ( 10.49211908931699178, -10.00000000000000000, -5.000000000000000000 ) ) ;
#9097=CARTESIAN_POINT ( 'NONE',  ( -46.99999999999998579, 65.00000000000000000, -12.50000000000000000 ) ) ;
#9103=CARTESIAN_POINT ( 'NONE',  ( -28.88216758755841695, 75.18040026313910573, -1.430629151363568718 ) ) ;
#9106=CIRCLE ( 'NONE', #12181, 14.99999999999999645 ) ;
#9112=CARTESIAN_POINT ( 'NONE',  ( -4.701390418375632763, 64.25000000000000000, 5.347094680480811490 ) ) ;
#9137=ORIENTED_EDGE ( 'NONE', *, *, #8901, .T. ) ;
#9140=CARTESIAN_POINT ( 'NONE',  ( -11.51245442718898992, 12.87030402641002702, 11.66749078037026521 ) ) ;
#9142=VECTOR ( 'NONE', #12003, 1000.000000000000000 ) ;
#9153=ORIENTED_EDGE ( 'NONE', *, *, #19437, .T. ) ;
#9162=CARTESIAN_POINT ( 'NONE',  ( 45.00000000000000000, -10.00000000000000000, 0.000000000000000000 ) ) ;
#9178=CARTESIAN_POINT ( 'NONE',  ( -20.76827921581725178, 50.35794673965182966, -15.75863071056655329 ) ) ;
#9186=DIRECTION ( 'NONE',  ( 0.000000000000000000, 0.000000000000000000, -1.000000000000000000 ) ) ;
#9188=CARTESIAN_POINT ( 'NONE',  ( -3.532373732925984111, 79.99999999989431387, -0.9530258780636241545 ) ) ;
#9192=CARTESIAN_POINT ( 'NONE',  ( -14.99999999999999645, 5.000000000000000000, 30.00000000000000000 ) ) ;
#9193=CARTESIAN_POINT ( 'NONE',  ( -27.89607850596237171, 49.99668640821654719, -12.77299574469434518 ) ) ;
#9194=CARTESIAN_POINT ( 'NONE',  ( -27.75180011566605742, 9.360503832615256314, -4.272254040061502778 ) ) ;
#9196=AXIS2_PLACEMENT_3D ( 'NONE', #11064, #3008, #6579 ) ;
#9209=VERTEX_POINT ( 'NONE', #6415 ) ;
#9214=VECTOR ( 'NONE', #1509, 1000.000000000000000 ) ;
#9219=CARTESIAN_POINT ( 'NONE',  ( -1.799176528135633335, 64.25000000000000000, 2.745993778453641010 ) ) ;
#9224=DIRECTION ( 'NONE',  ( 0.000000000000000000, 0.000000000000000000, -1.000000000000000000 ) ) ;
#9226=AXIS2_PLACEMENT_3D ( 'NONE', #1353, #17571, #12907 ) ;
#9227=FACE_OUTER_BOUND ( 'NONE', #9337, .T. ) ;
#9229=EDGE_CURVE ( 'NONE', #5484, #7189, #11839, .T. ) ;
#9239=CARTESIAN_POINT ( 'NONE',  ( -15.99999999999999289, 20.09941697557067997, 4.999999999999989342 ) ) ;
#9245=CARTESIAN_POINT ( 'NONE',  ( -15.99999999999999289, 65.74999999999998579, 0.000000000000000000 ) ) ;
#9247=EDGE_CURVE ( 'NONE', #17344, #8219, #6383, .T. ) ;
#9258=DIRECTION ( 'NONE',  ( 0.000000000000000000, -1.000000000000000000, 0.000000000000000000 ) ) ;
#9268=CARTESIAN_POINT ( 'NONE',  ( -20.99999999999998224, 15.09941697557068530, 11.45643923738960446 ) ) ;
#9279=CARTESIAN_POINT ( 'NONE',  ( -16.69844302412945325, 45.63488619083994990, -12.49945479904454437 ) ) ;
#9293=CARTESIAN_POINT ( 'NONE',  ( -0.9949668995500261515, 50.22606426727399054, -9.888289806186126185 ) ) ;
#9294=CARTESIAN_POINT ( 'NONE',  ( -28.42825495836414618, 8.666880057480497612, -1.380138809628029595 ) ) ;
#9306=CARTESIAN_POINT ( 'NONE',  ( -20.48867580399955202, 17.32628949019004594, 11.66705517935763936 ) ) ;
#9317=CARTESIAN_POINT ( 'NONE',  ( -3.876681006550094288, 75.90505089109430514, 3.056606027154308514 ) ) ;
#9334=CARTESIAN_POINT ( 'NONE',  ( 10.49211908931699178, -10.00000000000000000, 0.000000000000000000 ) ) ;
#9337=EDGE_LOOP ( 'NONE', ( #16565, #7389, #20220, #9599, #3846, #9773, #7970, #9053 ) ) ;
#9352=DIRECTION ( 'NONE',  ( -1.000000000000000000, 0.000000000000000000, 0.000000000000000000 ) ) ;
#9353=DIRECTION ( 'NONE',  ( 0.000000000000000000, 0.000000000000000000, 1.000000000000000000 ) ) ;
#9359=DIRECTION ( 'NONE',  ( 0.000000000000000000, -1.000000000000000000, 0.000000000000000000 ) ) ;
#9382=CARTESIAN_POINT ( 'NONE',  ( -7.293433234389345543, 44.99741180067891122, -8.975862722551676498 ) ) ;
#9386=CARTESIAN_POINT ( 'NONE',  ( -21.92567948885827178, 45.20990627917875315, -11.03350026938877093 ) ) ;
#9388=ORIENTED_EDGE ( 'NONE', *, *, #7327, .T. ) ;
#9393=CARTESIAN_POINT ( 'NONE',  ( 1.469533291826635724, 76.75544209469038037, -3.174647668802506484 ) ) ;
#9394=ORIENTED_EDGE ( 'NONE', *, *, #14243, .T. ) ;
#9397=CARTESIAN_POINT ( 'NONE',  ( -15.99999999999999289, 80.00000000000000000, 0.000000000000000000 ) ) ;
#9399=CARTESIAN_POINT ( 'NONE',  ( -19.92414059662587533, 50.39646155737152355, -15.92985716015406972 ) ) ;
#9402=EDGE_CURVE ( 'NONE', #20090, #17792, #2722, .T. ) ;
#9410=CARTESIAN_POINT ( 'NONE',  ( -11.00000000000000355, 15.09941697557068530, 11.45643923738960446 ) ) ;
#9415=CARTESIAN_POINT ( 'NONE',  ( -27.42006910542679776, 68.94695149080686747, 5.083831496961733976 ) ) ;
#9418=DIRECTION ( 'NONE',  ( 1.000000000000000000, 0.000000000000000000, 0.000000000000000000 ) ) ;
#9426=CARTESIAN_POINT ( 'NONE',  ( 0.6802973005055915623, 71.85025536417184355, 0.8468720397213821416 ) ) ;
#9428=CARTESIAN_POINT ( 'NONE',  ( -20.63965592820711237, 79.99566203514093843, -12.08264426539709468 ) ) ;
#9433=DIRECTION ( 'NONE',  ( 0.000000000000000000, -0.000000000000000000, 1.000000000000000000 ) ) ;
#9443=EDGE_LOOP ( 'NONE', ( #19381, #6303, #810, #3517 ) ) ;
#9451=VERTEX_POINT ( 'NONE', #17664 ) ;
#9458=CARTESIAN_POINT ( 'NONE',  ( -30.58332872481887321, 79.14063577707173636, -7.486051927416412788 ) ) ;
#9474=CARTESIAN_POINT ( 'NONE',  ( -35.00000000000000000, 64.25000000000000000, 75.00000000000000000 ) ) ;
#9476=AXIS2_PLACEMENT_3D ( 'NONE', #8950, #3101, #14061 ) ;
#9477=ADVANCED_FACE ( 'NONE', ( #372 ), #16474, .T. ) ;
#9478=DIRECTION ( 'NONE',  ( -0.000000000000000000, 1.000000000000000000, -0.000000000000000000 ) ) ;
#9489=CARTESIAN_POINT ( 'NONE',  ( -5.931730174668158106, 45.09262939792821356, -7.439426869663584796 ) ) ;
#9494=CARTESIAN_POINT ( 'NONE',  ( -20.16417779879374450, 45.40494962656599398, -11.79224875690949759 ) ) ;
#9496=VERTEX_POINT ( 'NONE', #17871 ) ;
#9498=ORIENTED_EDGE ( 'NONE', *, *, #20128, .T. ) ;
#9501=CARTESIAN_POINT ( 'NONE',  ( -10.87002103192357616, 79.99099046118973888, -11.97147087691752532 ) ) ;
#9503=ORIENTED_EDGE ( 'NONE', *, *, #5834, .T. ) ;
#9520=CARTESIAN_POINT ( 'NONE',  ( -28.72613570046926768, 61.69439188727080392, 2.139313856061467511 ) ) ;
#9521=LINE ( 'NONE', #4864, #7209 ) ;
#9523=DIRECTION ( 'NONE',  ( 0.000000000000000000, 0.000000000000000000, -1.000000000000000000 ) ) ;
#9531=ORIENTED_EDGE ( 'NONE', *, *, #3208, .T. ) ;
#9536=CARTESIAN_POINT ( 'NONE',  ( -29.92243289137827134, 79.32232495077528256, -8.031676520616485959 ) ) ;
#9542=FACE_OUTER_BOUND ( 'NONE', #8095, .T. ) ;
#9551=CARTESIAN_POINT ( 'NONE',  ( -11.00000000000000355, 15.09941697557068530, 11.45643923738960446 ) ) ;
#9555=CARTESIAN_POINT ( 'NONE',  ( -11.59722103597593801, 18.53029315133363752, 3.430876175762952673 ) ) ;
#9570=CARTESIAN_POINT ( 'NONE',  ( -26.44938323691329884, 79.57013539180375972, -8.777265990090930003 ) ) ;
#9575=DIRECTION ( 'NONE',  ( 0.000000000000000000, 0.000000000000000000, 1.000000000000000000 ) ) ;
#9585=CARTESIAN_POINT ( 'NONE',  ( 10.49211908931699178, 5.000000000000000000, 0.000000000000000000 ) ) ;
#9587=CARTESIAN_POINT ( 'NONE',  ( -30.00000000000005329, 4.999999999999980460, -7.692611737894555546 ) ) ;
#9589=ORIENTED_EDGE ( 'NONE', *, *, #20551, .F. ) ;
#9593=CARTESIAN_POINT ( 'NONE',  ( 10.49211908931699178, -10.00000000000000000, 5.999999999999998224 ) ) ;
#9594=CARTESIAN_POINT ( 'NONE',  ( -5.369514813894758376, 45.26689869013502232, -6.584760213112335947 ) ) ;
#9597=ADVANCED_FACE ( 'NONE', ( #6597 ), #1747, .T. ) ;
#9598=CARTESIAN_POINT ( 'NONE',  ( -26.45282069710705386, 45.18437375736277062, -6.897582699900483227 ) ) ;
#9599=ORIENTED_EDGE ( 'NONE', *, *, #9858, .T. ) ;
#9606=CARTESIAN_POINT ( 'NONE',  ( -8.197862634022071049, 79.89664383654030644, -10.58772689523680377 ) ) ;
#9624=CARTESIAN_POINT ( 'NONE',  ( -28.76203598978908005, 60.93597901302553055, 1.948583232574534696 ) ) ;
#9625=CARTESIAN_POINT ( 'NONE',  ( -15.99999999999999289, 80.00000000000000000, 4.999999999999989342 ) ) ;
#9627=DIRECTION ( 'NONE',  ( 0.000000000000000000, 0.000000000000000000, 1.000000000000000000 ) ) ;
#9631=VERTEX_POINT ( 'NONE', #7238 ) ;
#9634=ORIENTED_EDGE ( 'NONE', *, *, #14045, .T. ) ;
#9636=CARTESIAN_POINT ( 'NONE',  ( 0.3880700646982117585, 70.47620764902606538, 1.501429235142761609 ) ) ;
#9645=PLANE ( 'NONE',  #16220 ) ;
#9652=CARTESIAN_POINT ( 'NONE',  ( 30.10683012259193703, 0.000000000000000000, 5.999999999999998224 ) ) ;
#9655=AXIS2_PLACEMENT_3D ( 'NONE', #655, #11899, #2572 ) ;
#9659=FACE_OUTER_BOUND ( 'NONE', #10142, .T. ) ;
#9663=CARTESIAN_POINT ( 'NONE',  ( 45.00000000000000000, 5.000000000000000000, -15.00000000000000000 ) ) ;
#9664=FACE_OUTER_BOUND ( 'NONE', #15225, .T. ) ;
#9665=VERTEX_POINT ( 'NONE', #2063 ) ;
#9666=VERTEX_POINT ( 'NONE', #476 ) ;
#9677=DIRECTION ( 'NONE',  ( 1.000000000000000000, 0.000000000000000000, -0.000000000000000000 ) ) ;
#9678=ORIENTED_EDGE ( 'NONE', *, *, #17292, .T. ) ;
#9690=DIRECTION ( 'NONE',  ( 0.03124427847888152504, -0.6611148994991491445, 0.7496338337632341142 ) ) ;
#9691=CARTESIAN_POINT ( 'NONE',  ( -28.06779644517114036, 9.091084443369014778, -3.324986922928176547 ) ) ;
#9697=CARTESIAN_POINT ( 'NONE',  ( -5.193025761855540878, 45.33914674468751116, -6.290980308501477936 ) ) ;
#9703=ORIENTED_EDGE ( 'NONE', *, *, #7190, .T. ) ;
#9707=CARTESIAN_POINT ( 'NONE',  ( -7.003725213616844414, 79.78781110430779222, -9.858226064142291634 ) ) ;
#9714=CARTESIAN_POINT ( 'NONE',  ( -32.50512987981172586, 58.97167237099849757, 1.240746080457016509 ) ) ;
#9724=CARTESIAN_POINT ( 'NONE',  ( -27.94575092597936816, 55.59861081455196086, 3.685053742613256578 ) ) ;
#9730=PLANE ( 'NONE',  #11159 ) ;
#9732=ADVANCED_FACE ( 'NONE', ( #10408 ), #3740, .F. ) ;
#9743=ORIENTED_EDGE ( 'NONE', *, *, #3189, .T. ) ;
#9753=AXIS2_PLACEMENT_3D ( 'NONE', #16057, #11158, #6266 ) ;
#9755=VERTEX_POINT ( 'NONE', #20273 ) ;
#9763=ORIENTED_EDGE ( 'NONE', *, *, #10274, .T. ) ;
#9766=DIRECTION ( 'NONE',  ( 0.000000000000000000, 0.000000000000000000, -1.000000000000000000 ) ) ;
#9770=CARTESIAN_POINT ( 'NONE',  ( -32.70858515791243093, 78.02673419565032020, -5.061054382488067382 ) ) ;
#9772=EDGE_CURVE ( 'NONE', #3281, #11977, #18693, .T. ) ;
#9773=ORIENTED_EDGE ( 'NONE', *, *, #15373, .T. ) ;
#9774=CARTESIAN_POINT ( 'NONE',  ( -15.99999999999999289, 9.999999999999994671, 12.50000000000000000 ) ) ;
#9792=CARTESIAN_POINT ( 'NONE',  ( 10.49211908931699178, -10.00000000000000000, 0.000000000000000000 ) ) ;
#9798=CARTESIAN_POINT ( 'NONE',  ( -4.411380774409790817, 58.90144870373934083, 4.688306218574344264 ) ) ;
#9799=VECTOR ( 'NONE', #598, 1000.000000000000000 ) ;
#9802=CARTESIAN_POINT ( 'NONE',  ( -4.702552499873432268, 63.82970699952134197, 5.349554939795952535 ) ) ;
#9803=CARTESIAN_POINT ( 'NONE',  ( -15.06548238822073671, 80.00001702854306984, -12.48688330620196929 ) ) ;
#9818=VECTOR ( 'NONE', #8403, 1000.000000000000000 ) ;
#9828=AXIS2_PLACEMENT_3D ( 'NONE', #8010, #5043, #19460 ) ;
#9831=CARTESIAN_POINT ( 'NONE',  ( 28.00000000000001066, 65.75000000000001421, 1.479896280015810639 ) ) ;
#9851=CARTESIAN_POINT ( 'NONE',  ( -28.99999999999999289, 0.000000000000000000, -15.00000000000000000 ) ) ;
#9858=EDGE_CURVE ( 'NONE', #1521, #20014, #1107, .T. ) ;
#9881=DIRECTION ( 'NONE',  ( -0.000000000000000000, -1.000000000000000000, -0.000000000000000000 ) ) ;
#9892=DIRECTION ( 'NONE',  ( 0.000000000000000000, 0.000000000000000000, 1.000000000000000000 ) ) ;
#9899=EDGE_CURVE ( 'NONE', #8008, #1440, #553, .T. ) ;
#9903=CARTESIAN_POINT ( 'NONE',  ( -3.497189663385620761, 49.35567744637351240, -0.02171244038980547214 ) ) ;
#9910=DIRECTION ( 'NONE',  ( -0.000000000000000000, -0.000000000000000000, 1.000000000000000000 ) ) ;
#9914=CARTESIAN_POINT ( 'NONE',  ( -17.87065464597074893, 58.81735738840291106, -4.639596491434944348 ) ) ;
#9917=CARTESIAN_POINT ( 'NONE',  ( -16.00000000000007105, 58.38562172233837089, -4.999999999999997335 ) ) ;
#9926=EDGE_CURVE ( 'NONE', #20835, #19075, #5795, .T. ) ;
#9928=CARTESIAN_POINT ( 'NONE',  ( -28.68049345341341194, 53.83925212050883857, -2.471093196081551646 ) ) ;
#9933=DIRECTION ( 'NONE',  ( 1.000000000000000000, 0.000000000000000000, 0.000000000000000000 ) ) ;
#9938=CARTESIAN_POINT ( 'NONE',  ( -4.702542490863385716, 65.65291453363785479, 5.349528374469380232 ) ) ;
#9942=CARTESIAN_POINT ( 'NONE',  ( -28.94448814640270129, 65.74999999999995737, 3.385962996190683860 ) ) ;
#9956=CARTESIAN_POINT ( 'NONE',  ( -15.81957430612866311, 71.61437827766145858, -4.999999999999988454 ) ) ;
#9966=CARTESIAN_POINT ( 'NONE',  ( -21.63278055428463276, 79.98685641808557989, -11.85964839587038000 ) ) ;
#9971=CIRCLE ( 'NONE', #8646, 9.999999999999998224 ) ;
#9979=EDGE_CURVE ( 'NONE', #2271, #8514, #8861, .T. ) ;
#9980=CIRCLE ( 'NONE', #19470, 13.99999999999999822 ) ;
#9992=VECTOR ( 'NONE', #14813, 1000.000000000000000 ) ;
#9995=VERTEX_POINT ( 'NONE', #13894 ) ;
#9998=CARTESIAN_POINT ( 'NONE',  ( 1.503934470862336559, 53.26675808472690932, -3.147798062369893124 ) ) ;
#9999=CARTESIAN_POINT ( 'NONE',  ( -15.99999999999999289, 9.999999999999994671, -17.50000000000000000 ) ) ;
#10015=CARTESIAN_POINT ( 'NONE',  ( -16.88984037207102062, 58.47342245001757277, -4.923257761629218798 ) ) ;
#10017=CARTESIAN_POINT ( 'NONE',  ( -15.81983077554147421, 58.38562172233856273, -4.999999999999992895 ) ) ;
#10027=CARTESIAN_POINT ( 'NONE',  ( -28.90575499228997103, 55.17197461462945540, -1.140010367715231343 ) ) ;
#10028=CARTESIAN_POINT ( 'NONE',  ( -18.65171524015568139, 19.34141692181273342, 12.21627542118126541 ) ) ;
#10029=EDGE_CURVE ( 'NONE', #3306, #4564, #12934, .T. ) ;
#10031=LINE ( 'NONE', #13141, #8321 ) ;
#10038=ORIENTED_EDGE ( 'NONE', *, *, #11869, .F. ) ;
#10047=CARTESIAN_POINT ( 'NONE',  ( -30.87525101170383124, 65.74999999999997158, 2.549678278787586461 ) ) ;
#10056=FACE_OUTER_BOUND ( 'NONE', #1362, .T. ) ;
#10076=CARTESIAN_POINT ( 'NONE',  ( -24.99627478638403844, 79.78781110430777801, -9.858226064141845768 ) ) ;
#10080=AXIS2_PLACEMENT_3D ( 'NONE', #15484, #12706, #18753 ) ;
#10081=DIRECTION ( 'NONE',  ( 1.000000000000000000, 0.000000000000000000, 0.000000000000000000 ) ) ;
#10084=CARTESIAN_POINT ( 'NONE',  ( -15.99999999999999289, 80.00000000000000000, -4.999999999999989342 ) ) ;
#10089=CARTESIAN_POINT ( 'NONE',  ( -7.939600225062636518, 79.94564677075823056, -11.17290160265476473 ) ) ;
#10097=CARTESIAN_POINT ( 'NONE',  ( -29.99999999999979039, 5.000000000000201617, 0.4679281238166860257 ) ) ;
#10103=CARTESIAN_POINT ( 'NONE',  ( -7.000292895910345869, 44.98883621322416104, -8.709882378375517931 ) ) ;
#10104=AXIS2_PLACEMENT_3D ( 'NONE', #12511, #18557, #5817 ) ;
#10105=ORIENTED_EDGE ( 'NONE', *, *, #8614, .F. ) ;
#10107=CARTESIAN_POINT ( 'NONE',  ( -3.048040018689400110, 56.82851019708963491, 0.1106114228930126370 ) ) ;
#10110=CARTESIAN_POINT ( 'NONE',  ( -15.99999999999999289, 80.00000000000000000, -12.50000000000000000 ) ) ;
#10113=ORIENTED_EDGE ( 'NONE', *, *, #4437, .F. ) ;
#10117=EDGE_CURVE ( 'NONE', #1421, #10783, #2096, .T. ) ;
#10131=CARTESIAN_POINT ( 'NONE',  ( -28.48657445126280763, 48.50183867280838257, -0.8242875664313024098 ) ) ;
#10141=AXIS2_PLACEMENT_3D ( 'NONE', #6916, #8829, #5536 ) ;
#10142=EDGE_LOOP ( 'NONE', ( #15612, #4054, #4509 ) ) ;
#10160=EDGE_CURVE ( 'NONE', #7321, #8661, #14009, .T. ) ;
#10166=CARTESIAN_POINT ( 'NONE',  ( -1.115519630330159551, 65.75000000000000000, 2.547625675852271510 ) ) ;
#10169=CARTESIAN_POINT ( 'NONE',  ( -12.70096667698038928, 69.85981968218749216, -3.758841495318840042 ) ) ;
#10173=ORIENTED_EDGE ( 'NONE', *, *, #12429, .T. ) ;
#10197=CARTESIAN_POINT ( 'NONE',  ( -2.899236859673289146, 78.36047030499231880, -5.510874449651578466 ) ) ;
#10208=CARTESIAN_POINT ( 'NONE',  ( -26.75565744063416318, 9.893465008606606048, 6.378074558502260238 ) ) ;
#10213=CARTESIAN_POINT ( 'NONE',  ( -3.927421424228952684, 54.52359887367414615, 3.254349035475716967 ) ) ;
#10216=CARTESIAN_POINT ( 'NONE',  ( -4.579482833895355931, 60.98411661173300047, 5.082820002145302496 ) ) ;
#10217=CARTESIAN_POINT ( 'NONE',  ( -3.572474243005702821, 79.61902841131316677, -9.096985201275369803 ) ) ;
#10223=ORIENTED_EDGE ( 'NONE', *, *, #20711, .T. ) ;
#10241=CARTESIAN_POINT ( 'NONE',  ( -31.15489049490080475, 50.26056083818948395, -9.697909921291566704 ) ) ;
#10256=ORIENTED_EDGE ( 'NONE', *, *, #7335, .F. ) ;
#10274=EDGE_CURVE ( 'NONE', #6959, #15695, #3171, .T. ) ;
#10281=EDGE_LOOP ( 'NONE', ( #7311, #4692, #18086, #15251 ) ) ;
#10287=CARTESIAN_POINT ( 'NONE',  ( -25.37873435132391009, 79.74334935823260651, -9.599827418924029132 ) ) ;
#10291=DIRECTION ( 'NONE',  ( 0.000000000000000000, 0.000000000000000000, -1.000000000000000000 ) ) ;
#10297=DIRECTION ( 'NONE',  ( -0.000000000000000000, 1.000000000000000000, -0.000000000000000000 ) ) ;
#10304=CYLINDRICAL_SURFACE ( 'NONE', #17332, 5.999999999999998224 ) ;
#10306=CARTESIAN_POINT ( 'NONE',  ( -0.1767699604045824824, 65.74999999999997158, 2.481238266578629226 ) ) ;
#10311=CARTESIAN_POINT ( 'NONE',  ( -29.99999999999999645, 5.000000000000000000, 10.50000000000000711 ) ) ;
#10317=DIRECTION ( 'NONE',  ( 1.000000000000000000, 0.000000000000000000, 0.000000000000000000 ) ) ;
#10321=CARTESIAN_POINT ( 'NONE',  ( -0.1881451998551312010, 64.85124100632805266, 2.499262340588669584 ) ) ;
#10324=CARTESIAN_POINT ( 'NONE',  ( -34.00000000000000711, 64.25000000000000000, 2.481238266578627449 ) ) ;
#10343=VECTOR ( 'NONE', #6144, 1000.000000000000000 ) ;
#10348=CARTESIAN_POINT ( 'NONE',  ( -26.82492178207555611, 45.34741445055429665, -6.259914210700230797 ) ) ;
#10375=FACE_OUTER_BOUND ( 'NONE', #5902, .T. ) ;
#10390=CARTESIAN_POINT ( 'NONE',  ( -17.04169990913787913, 79.99999999999985789, -12.45923801546573095 ) ) ;
#10394=ADVANCED_FACE ( 'NONE', ( #18533 ), #20212, .F. ) ;
#10401=CARTESIAN_POINT ( 'NONE',  ( -27.29860958162435480, 64.25000000000000000, 5.347094680480811490 ) ) ;
#10408=FACE_OUTER_BOUND ( 'NONE', #8989, .T. ) ;
#10410=ORIENTED_EDGE ( 'NONE', *, *, #8777, .T. ) ;
#10416=ADVANCED_FACE ( 'NONE', ( #20009 ), #725, .T. ) ;
#10419=CARTESIAN_POINT ( 'NONE',  ( -29.99999999999966249, 5.000000000000310862, 0.9384178472467484822 ) ) ;
#10439=FACE_OUTER_BOUND ( 'NONE', #2405, .T. ) ;
#10447=CARTESIAN_POINT ( 'NONE',  ( -16.71219703957330438, 71.55985624430604730, -4.952210724505382800 ) ) ;
#10452=CARTESIAN_POINT ( 'NONE',  ( -25.97610854243320588, 50.06551567652685009, -13.91464430999257651 ) ) ;
#10455=CARTESIAN_POINT ( 'NONE',  ( -28.30706676095798713, 52.46230133324129952, 2.217793569358140537 ) ) ;
#10480=AXIS2_PLACEMENT_3D ( 'NONE', #5315, #368, #19749 ) ;
#10481=CARTESIAN_POINT ( 'NONE',  ( -27.91449807164519825, 74.13367381892543051, 3.782735275914649087 ) ) ;
#10496=DIRECTION ( 'NONE',  ( 0.5999999999999998668, 2.775557561562894309E-16, -0.8000000000000001554 ) ) ;
#10507=VECTOR ( 'NONE', #17228, 1000.000000000000000 ) ;
#10510=CARTESIAN_POINT ( 'NONE',  ( -27.76586288966045046, 64.25000000000001421, 4.519411796990929098 ) ) ;
#10517=CARTESIAN_POINT ( 'NONE',  ( -15.73951718899008512, 80.00000000000179057, -12.49947570859690416 ) ) ;
#10530=AXIS2_PLACEMENT_3D ( 'NONE', #2856, #15893, #6009 ) ;
#10536=DIRECTION ( 'NONE',  ( -0.000000000000000000, -0.000000000000000000, 1.000000000000000000 ) ) ;
#10554=VERTEX_POINT ( 'NONE', #7594 ) ;
#10558=CARTESIAN_POINT ( 'NONE',  ( 30.00000000000000000, -10.00000000000000000, 15.00000000000000000 ) ) ;
#10559=DIRECTION ( 'NONE',  ( 0.000000000000000000, -1.000000000000000000, 0.000000000000000000 ) ) ;
#10560=CARTESIAN_POINT ( 'NONE',  ( -18.30887993796372726, 70.93184341055301445, -4.446547635559178424 ) ) ;
#10561=EDGE_CURVE ( 'NONE', #491, #6727, #2633, .T. ) ;
#10567=CARTESIAN_POINT ( 'NONE',  ( -19.40591372560455596, 45.47726231970822397, -12.03202924821253283 ) ) ;
#10581=CARTESIAN_POINT ( 'NONE',  ( -0.7537384908010169582, 50.28366646829528719, -9.578226701023302425 ) ) ;
#10584=VERTEX_POINT ( 'NONE', #19056 ) ;
#10589=CARTESIAN_POINT ( 'NONE',  ( -20.89897948556633978, 16.09941697557071905, 0.9999999999999991118 ) ) ;
#10619=PLANE ( 'NONE',  #20910 ) ;
#10630=VERTEX_POINT ( 'NONE', #9593 ) ;
#10641=CYLINDRICAL_SURFACE ( 'NONE', #253, 15.00000000000000000 ) ;
#10654=CARTESIAN_POINT ( 'NONE',  ( -20.31374355284814825, 65.74999999999995737, -2.528164662410434804 ) ) ;
#10664=CARTESIAN_POINT ( 'NONE',  ( -14.07807032132161318, 50.45729534307898234, -16.17568974221241618 ) ) ;
#10666=VECTOR ( 'NONE', #12649, 1000.000000000000000 ) ;
#10668=CARTESIAN_POINT ( 'NONE',  ( -28.49367486532711524, 49.92396641514135069, 0.4641840246318328922 ) ) ;
#10673=CARTESIAN_POINT ( 'NONE',  ( -3.513138912839586681, 80.00000000007391066, -0.6469719004569252085 ) ) ;
#10674=ORIENTED_EDGE ( 'NONE', *, *, #6765, .F. ) ;
#10675=ORIENTED_EDGE ( 'NONE', *, *, #18062, .T. ) ;
#10679=CARTESIAN_POINT ( 'NONE',  ( -2.305711553939125746, 50.03762982245009283, -11.32446199378746421 ) ) ;
#10680=CARTESIAN_POINT ( 'NONE',  ( -33.99999999999997868, 65.74999999999995737, -2.528164662410434804 ) ) ;
#10699=CARTESIAN_POINT ( 'NONE',  ( -28.94934366394663883, 73.64887869707766299, -0.2211343278575746418 ) ) ;
#10708=EDGE_CURVE ( 'NONE', #5066, #15695, #5159, .T. ) ;
#10716=ORIENTED_EDGE ( 'NONE', *, *, #8492, .T. ) ;
#10718=DIRECTION ( 'NONE',  ( -0.000000000000000000, -1.000000000000000000, -0.000000000000000000 ) ) ;
#10720=CARTESIAN_POINT ( 'NONE',  ( -29.99999999999999645, 5.000000000000000000, 30.00000000000000000 ) ) ;
#10724=DIRECTION ( 'NONE',  ( 0.000000000000000000, 0.000000000000000000, 1.000000000000000000 ) ) ;
#10731=CARTESIAN_POINT ( 'NONE',  ( -15.73952097860949273, 79.99999999999998579, -12.49895143242785345 ) ) ;
#10735=CARTESIAN_POINT ( 'NONE',  ( -15.99999999999999289, 10.09941697557069418, 12.50000000000000000 ) ) ;
#10756=ORIENTED_EDGE ( 'NONE', *, *, #9073, .T. ) ;
#10760=CARTESIAN_POINT ( 'NONE',  ( -20.83678142705256064, 13.78956489930263452, 11.52651691409252521 ) ) ;
#10768=ORIENTED_EDGE ( 'NONE', *, *, #11932, .T. ) ;
#10770=B_SPLINE_CURVE_WITH_KNOTS ( 'NONE', 3,
 ( #11831, #16493, #9803, #14720, #1974, #14824, #17888, #388, #19665, #19872, #3655, #18291, #6840, #3765, #10217, #8538, #15039, #16711, #14923, #4935, #13324, #174, #497, #19452, #2189, #19771, #6514, #5237, #11728, #8641, #18190, #6936 ),
 .UNSPECIFIED., .F., .F.,
 ( 4, 2, 2, 2, 2, 2, 2, 2, 2, 2, 2, 2, 2, 2, 2, 4 ),
 ( -0.0002012768826452384079, 0.001195388216070833671, 0.002592053314786905722, 0.005385383512219049824, 0.008178713709651194361, 0.009575378808367264460, 0.01097204390708333629, 0.01376537410451547823, 0.01516203920323155353, 0.01655870430194762363, 0.01795536940066369894, 0.01865370195002173312, 0.01935203449937976730, 0.02074869959809586342, 0.02144703214745389760, 0.02214536469681193526 ),
 .UNSPECIFIED. ) ;
#10772=CARTESIAN_POINT ( 'NONE',  ( -29.99999999999999645, -10.00000000000000000, 0.000000000000000000 ) ) ;
#10773=CARTESIAN_POINT ( 'NONE',  ( -22.54565399147047344, 45.14475518768605866, -10.65478537919073254 ) ) ;
#10777=CARTESIAN_POINT ( 'NONE',  ( -28.15715448389819997, 53.81647424313067773, 2.930203991123683238 ) ) ;
#10783=VERTEX_POINT ( 'NONE', #7062 ) ;
#10784=ORIENTED_EDGE ( 'NONE', *, *, #10160, .T. ) ;
#10787=CARTESIAN_POINT ( 'NONE',  ( -17.58792505510971083, 50.46559566222132531, -16.20915785584423929 ) ) ;
#10799=EDGE_CURVE ( 'NONE', #17847, #245, #11659, .T. ) ;
#10802=DIRECTION ( 'NONE',  ( -0.000000000000000000, -1.000000000000000000, -0.000000000000000000 ) ) ;
#10803=CARTESIAN_POINT ( 'NONE',  ( -28.65583546987735275, 66.09831342192320847, 2.470462955490114965 ) ) ;
#10806=AXIS2_PLACEMENT_3D ( 'NONE', #18531, #8872, #14084 ) ;
#10814=VECTOR ( 'NONE', #20796, 1000.000000000000000 ) ;
#10822=DIRECTION ( 'NONE',  ( 0.000000000000000000, -1.000000000000000000, 0.000000000000000000 ) ) ;
#10823=CARTESIAN_POINT ( 'NONE',  ( -25.99999999999999645, 9.999999999999994671, -7.500000000000000000 ) ) ;
#10845=AXIS2_PLACEMENT_3D ( 'NONE', #16951, #8786, #11980 ) ;
#10846=LINE ( 'NONE', #2813, #19499 ) ;
#10847=LINE ( 'NONE', #4290, #262 ) ;
#10870=CARTESIAN_POINT ( 'NONE',  ( -15.99999999999999289, 10.09941697557069418, 12.50000000000000000 ) ) ;
#10877=CIRCLE ( 'NONE', #11903, 5.999999999999998224 ) ;
#10881=DIRECTION ( 'NONE',  ( 0.000000000000000000, 0.000000000000000000, 1.000000000000000000 ) ) ;
#10882=CARTESIAN_POINT ( 'NONE',  ( -19.64325535697088654, 49.51382188615453117, -11.96543228433093198 ) ) ;
#10900=CARTESIAN_POINT ( 'NONE',  ( -22.23810050820787865, 50.28853357967717130, -15.44648544901684950 ) ) ;
#10901=FACE_OUTER_BOUND ( 'NONE', #17472, .T. ) ;
#10902=ORIENTED_EDGE ( 'NONE', *, *, #9926, .T. ) ;
#10908=AXIS2_PLACEMENT_3D ( 'NONE', #2711, #12569, #10968 ) ;
#10928=ORIENTED_EDGE ( 'NONE', *, *, #13, .T. ) ;
#10930=ORIENTED_EDGE ( 'NONE', *, *, #10274, .F. ) ;
#10931=CARTESIAN_POINT ( 'NONE',  ( -3.074305435089455862, 72.33610889977832414, 0.5975377147116670562 ) ) ;
#10937=DIRECTION ( 'NONE',  ( 1.000000000000000000, -0.000000000000000000, -0.000000000000000000 ) ) ;
#10943=LINE ( 'NONE', #7751, #10666 ) ;
#10952=CARTESIAN_POINT ( 'NONE',  ( -4.693238136585347497, 66.39265442260773398, 5.329868606387891283 ) ) ;
#10956=CARTESIAN_POINT ( 'NONE',  ( -28.62307079896444506, 76.35052269458219598, -2.692414605357462687 ) ) ;
#10961=CARTESIAN_POINT ( 'NONE',  ( -13.77473633848136636, 10.61006857860113151, 12.30409397790407233 ) ) ;
#10965=CARTESIAN_POINT ( 'NONE',  ( 45.00000000000000000, 5.000000000000000000, 15.00000000000000000 ) ) ;
#10968=DIRECTION ( 'NONE',  ( 0.000000000000000000, 0.000000000000000000, -1.000000000000000000 ) ) ;
#10976=EDGE_CURVE ( 'NONE', #1421, #8955, #62, .T. ) ;
#10979=ORIENTED_EDGE ( 'NONE', *, *, #16868, .T. ) ;
#10997=CARTESIAN_POINT ( 'NONE',  ( -4.694333320860708980, 51.54365109033042103, -5.670238636117967523 ) ) ;
#11000=EDGE_CURVE ( 'NONE', #20919, #3253, #1793, .T. ) ;
#11002=CARTESIAN_POINT ( 'NONE',  ( -16.77277943456198628, 45.63508326896292999, -12.50000000000000178 ) ) ;
#11007=CARTESIAN_POINT ( 'NONE',  ( 0.7085851579124478050, 78.02673419564928281, -5.061054382486330105 ) ) ;
#11012=CARTESIAN_POINT ( 'NONE',  ( 1.349294741687074861, 52.07539629968670170, -4.877430129159401773 ) ) ;
#11013=DIRECTION ( 'NONE',  ( -1.000000000000000000, 0.000000000000000000, 0.000000000000000000 ) ) ;
#11024=CARTESIAN_POINT ( 'NONE',  ( -27.29860958162435480, 65.74999999999997158, 5.347094680480812379 ) ) ;
#11027=CARTESIAN_POINT ( 'NONE',  ( 27.33334827330880756, 65.75000000000001421, 2.147472525011945521 ) ) ;
#11035=CARTESIAN_POINT ( 'NONE',  ( 1.441635642453537702, 75.56468634061762657, -1.801359935164346115 ) ) ;
#11036=DIRECTION ( 'NONE',  ( 0.000000000000000000, 0.000000000000000000, -1.000000000000000000 ) ) ;
#11038=ORIENTED_EDGE ( 'NONE', *, *, #14210, .F. ) ;
#11045=CARTESIAN_POINT ( 'NONE',  ( 0.5040958584341809212, 58.95372983808996992, 1.249471100433037885 ) ) ;
#11055=DIRECTION ( 'NONE',  ( 0.000000000000000000, 0.000000000000000000, -1.000000000000000000 ) ) ;
#11060=CARTESIAN_POINT ( 'NONE',  ( -29.23300298503555439, 76.74099499729592821, -3.129240771529778975 ) ) ;
#11061=ORIENTED_EDGE ( 'NONE', *, *, #15108, .F. ) ;
#11063=CIRCLE ( 'NONE', #8690, 15.00000000000000000 ) ;
#11064=CARTESIAN_POINT ( 'NONE',  ( 30.00000000000000000, 0.000000000000000000, 15.00000000000000000 ) ) ;
#11065=EDGE_CURVE ( 'NONE', #14019, #12002, #8168, .T. ) ;
#11066=CARTESIAN_POINT ( 'NONE',  ( -33.44237801383309261, 75.57646748667876579, -1.814718499151628084 ) ) ;
#11072=EDGE_CURVE ( 'NONE', #15381, #1893, #14908, .T. ) ;
#11084=CARTESIAN_POINT ( 'NONE',  ( -19.31141590166239652, 11.33920243900448455, 12.05575761655145861 ) ) ;
#11085=DIRECTION ( 'NONE',  ( 0.000000000000000000, 0.000000000000000000, -1.000000000000000000 ) ) ;
#11087=ADVANCED_FACE ( 'NONE', ( #18389 ), #10304, .T. ) ;
#11088=CYLINDRICAL_SURFACE ( 'NONE', #16789, 4.999999999999989342 ) ;
#11089=AXIS2_PLACEMENT_3D ( 'NONE', #4750, #15704, #1372 ) ;
#11097=CARTESIAN_POINT ( 'NONE',  ( -8.542481363097889968, 50.20976409724571710, -15.00415514080579271 ) ) ;
#11105=CARTESIAN_POINT ( 'NONE',  ( -33.99999999999997868, 65.74999999999995737, -2.528164662410434804 ) ) ;
#11113=CARTESIAN_POINT ( 'NONE',  ( 30.10683012259193703, -24.14213562373095456, -4.999999999999997335 ) ) ;
#11119=EDGE_CURVE ( 'NONE', #15680, #9496, #482, .T. ) ;
#11136=CARTESIAN_POINT ( 'NONE',  ( -3.771940362451076556, 64.24999999999997158, 3.997049355788893976 ) ) ;
#11156=EDGE_CURVE ( 'NONE', #6192, #14773, #11926, .T. ) ;
#11158=DIRECTION ( 'NONE',  ( -0.000000000000000000, 1.000000000000000000, -0.000000000000000000 ) ) ;
#11159=AXIS2_PLACEMENT_3D ( 'NONE', #19390, #9933, #13247 ) ;
#11169=CARTESIAN_POINT ( 'NONE',  ( -26.55686023345718638, 79.99999999967671727, -6.747797645781123066 ) ) ;
#11174=B_SPLINE_CURVE_WITH_KNOTS ( 'NONE', 3,
 ( #1007, #7451, #20395, #5860 ),
 .UNSPECIFIED., .F., .F.,
 ( 4, 4 ),
 ( 0.000000000000000000, 0.001416029653785000168 ),
 .UNSPECIFIED. ) ;
#11185=EDGE_LOOP ( 'NONE', ( #19676, #8709, #15565, #12969 ) ) ;
#11194=CARTESIAN_POINT ( 'NONE',  ( -29.99999999999979039, 5.000000000000174971, -2.366409145735037800 ) ) ;
#11203=CARTESIAN_POINT ( 'NONE',  ( 0.3663305609645054473, 50.73190751614451699, -7.824425459317669862 ) ) ;
#11208=AXIS2_PLACEMENT_3D ( 'NONE', #2202, #3570, #13337 ) ;
#11215=CARTESIAN_POINT ( 'NONE',  ( -0.7874873115017846370, 78.92002130297213114, -6.902655774461555538 ) ) ;
#11218=EDGE_LOOP ( 'NONE', ( #13822, #14372, #16224, #1245 ) ) ;
#11229=( NAMED_UNIT ( * ) SI_UNIT ( $, .STERADIAN. ) SOLID_ANGLE_UNIT ( ) );
#11234=EDGE_CURVE ( 'NONE', #6984, #17847, #18448, .T. ) ;
#11237=CARTESIAN_POINT ( 'NONE',  ( -28.70953045725249453, 62.08313086074902287, 2.221255103732576064 ) ) ;
#11240=ORIENTED_EDGE ( 'NONE', *, *, #2378, .F. ) ;
#11241=CARTESIAN_POINT ( 'NONE',  ( -27.29745750913661340, 65.65291453363863639, 5.349528374469362468 ) ) ;
#11242=CARTESIAN_POINT ( 'NONE',  ( 10.49211908931699178, 5.000000000000000000, 0.000000000000000000 ) ) ;
#11247=AXIS2_PLACEMENT_3D ( 'NONE', #6372, #1729, #12869 ) ;
#11250=CARTESIAN_POINT ( 'NONE',  ( -3.810871963545228613, 76.46633113979204666, 2.786148689275818935 ) ) ;
#11251=CARTESIAN_POINT ( 'NONE',  ( 26.99999999999999645, 65.00000000000000000, -22.50000000000000000 ) ) ;
#11268=DIRECTION ( 'NONE',  ( -0.000000000000000000, -1.000000000000000000, -0.000000000000000000 ) ) ;
#11269=ORIENTED_EDGE ( 'NONE', *, *, #2524, .F. ) ;
#11288=CIRCLE ( 'NONE', #1813, 5.000000000000000888 ) ;
#11299=CARTESIAN_POINT ( 'NONE',  ( -26.09894814240073302, 5.223431272791994040, -7.368069150172500414 ) ) ;
#11303=EDGE_LOOP ( 'NONE', ( #20837, #13056, #4833, #18130, #448, #12926 ) ) ;
#11308=CARTESIAN_POINT ( 'NONE',  ( -3.810806528046885244, 49.99805885029708463, -12.54965585876388268 ) ) ;
#11313=EDGE_LOOP ( 'NONE', ( #10930, #9503, #10173, #737 ) ) ;
#11318=CARTESIAN_POINT ( 'NONE',  ( -12.40988168468657094, 79.99589872788176592, -12.11680902303699803 ) ) ;
#11320=VERTEX_POINT ( 'NONE', #13995 ) ;
#11321=ORIENTED_EDGE ( 'NONE', *, *, #5853, .T. ) ;
#11330=EDGE_CURVE ( 'NONE', #8514, #8072, #65, .T. ) ;
#11334=CARTESIAN_POINT ( 'NONE',  ( -28.87969541636898541, 58.77009191570905244, 1.174127190111078134 ) ) ;
#11341=ORIENTED_EDGE ( 'NONE', *, *, #162, .T. ) ;
#11344=EDGE_CURVE ( 'NONE', #9451, #9755, #15587, .T. ) ;
#11349=EDGE_CURVE ( 'NONE', #9995, #15623, #18678, .T. ) ;
#11357=CLOSED_SHELL ( 'NONE', ( #12534, #11087, #3022, #2912, #19772, #7314, #5729, #17829, #15025, #5257, #10394, #348, #4102, #17723, #4385, #2908, #18336, #1476, #3016, #6515, #10416, #8978, #17734, #4444, #1373, #3308, #20183, #11479, #14745, #5309, #72, #4094, #18634, #20603, #16136, #17077, #14806, #11631, #19399, #7295, #18109, #17914, #5100, #20024, #8332, #9732, #9597, #20055, #1269, #9477, #4501, #14503, #20688, #15731, #16359, #17431, #3676, #7482, #11371, #13573, #3947, #15758, #3548, #18413, #14769, #20663, #11645, #3577 ) ) ;
#11366=ORIENTED_EDGE ( 'NONE', *, *, #5970, .F. ) ;
#11371=ADVANCED_FACE ( 'NONE', ( #1263 ), #14101, .F. ) ;
#11374=CIRCLE ( 'NONE', #7972, 5.000000000000000000 ) ;
#11383=ORIENTED_EDGE ( 'NONE', *, *, #11065, .F. ) ;
#11397=DIRECTION ( 'NONE',  ( 0.000000000000000000, -1.000000000000000000, 0.000000000000000000 ) ) ;
#11400=CARTESIAN_POINT ( 'NONE',  ( -28.43128979000083234, 8.662912046624729356, -1.352006923338597177 ) ) ;
#11409=CARTESIAN_POINT ( 'NONE',  ( -9.201414108834393701, 49.63991447519583033, -10.51578306933696361 ) ) ;
#11412=CARTESIAN_POINT ( 'NONE',  ( -18.67450410742786815, 45.53668989701726133, -12.21661053328929469 ) ) ;
#11418=EDGE_LOOP ( 'NONE', ( #18778, #17564, #8253, #17644 ) ) ;
#11421=PLANE ( 'NONE',  #14644 ) ;
#11425=CARTESIAN_POINT ( 'NONE',  ( -11.68625644715183931, 64.25000000000000000, -2.528164662410438357 ) ) ;
#11449=ORIENTED_EDGE ( 'NONE', *, *, #1914, .F. ) ;
#11453=DIRECTION ( 'NONE',  ( 0.000000000000000000, 0.000000000000000000, -1.000000000000000000 ) ) ;
#11471=EDGE_CURVE ( 'NONE', #14019, #3348, #19447, .T. ) ;
#11473=EDGE_LOOP ( 'NONE', ( #6635, #2092 ) ) ;
#11478=CARTESIAN_POINT ( 'NONE',  ( -32.70485353615134017, 71.96725945621675180, 0.7929198755315589597 ) ) ;
#11479=ADVANCED_FACE ( 'NONE', ( #1989 ), #11421, .F. ) ;
#11496=FACE_OUTER_BOUND ( 'NONE', #8532, .T. ) ;
#11510=CARTESIAN_POINT ( 'NONE',  ( -3.102165542891348604, 55.17729803629858054, -1.148087882950909355 ) ) ;
#11523=CARTESIAN_POINT ( 'NONE',  ( -29.99999999999999645, 5.000000000000000000, 15.00000000000000000 ) ) ;
#11535=CIRCLE ( 'NONE', #11208, 4.999999999999997335 ) ;
#11538=CARTESIAN_POINT ( 'NONE',  ( -27.14901402057759938, 45.52498706128694295, -5.662591622423835069 ) ) ;
#11542=AXIS2_PLACEMENT_3D ( 'NONE', #7910, #6213, #9186 ) ;
#11552=TOROIDAL_SURFACE ( 'NONE', #11911, 17.50000000000000000, 5.000000000000000000 ) ;
#11558=VECTOR ( 'NONE', #13310, 1000.000000000000000 ) ;
#11560=CARTESIAN_POINT ( 'NONE',  ( -28.39840119452017575, 65.74999999999997158, 3.829763509598343330 ) ) ;
#11568=EDGE_LOOP ( 'NONE', ( #20899, #15586, #5253, #14472 ) ) ;
#11589=CARTESIAN_POINT ( 'NONE',  ( -20.99172629426764658, 79.99999999999126032, -11.47115151921912535 ) ) ;
#11590=AXIS2_PLACEMENT_3D ( 'NONE', #541, #13479, #5393 ) ;
#11614=CARTESIAN_POINT ( 'NONE',  ( -29.99999999999975842, 5.000000000000111022, -6.406390635520961219 ) ) ;
#11625=CARTESIAN_POINT ( 'NONE',  ( -3.512777538380836173, 50.29109887172522519, 0.7760323238818376268 ) ) ;
#11628=CARTESIAN_POINT ( 'NONE',  ( -33.48481952675158624, 76.25000000000001421, -2.578432583507804132 ) ) ;
#11631=ADVANCED_FACE ( 'NONE', ( #6072 ), #16662, .F. ) ;
#11638=VERTEX_POINT ( 'NONE', #19033 ) ;
#11639=CARTESIAN_POINT ( 'NONE',  ( -17.22997025788304271, 58.56006360057318005, -4.849479976237960344 ) ) ;
#11641=CARTESIAN_POINT ( 'NONE',  ( -11.86574742045090147, 62.48633020609619848, -2.814775708409676280 ) ) ;
#11642=CIRCLE ( 'NONE', #2501, 4.999999999999997335 ) ;
#11645=ADVANCED_FACE ( 'NONE', ( #17121 ), #9052, .T. ) ;
#11652=CARTESIAN_POINT ( 'NONE',  ( -33.12305221259295251, 56.12619721146663210, -0.3853563272486908997 ) ) ;
#11659=B_SPLINE_CURVE_WITH_KNOTS ( 'NONE', 3,
 ( #10870, #12583, #13862, #2726, #2831, #12477, #14184, #15674, #11084, #17138, #12689, #17240, #1139, #15567, #10760, #2624, #9066, #9268 ),
 .UNSPECIFIED., .F., .F.,
 ( 4, 2, 2, 2, 2, 2, 2, 2, 4 ),
 ( 0.007901880061100961111, 0.008888972354417348093, 0.009876064647733735075, 0.01086315694105012379, 0.01185024923436651077, 0.01283734152768289775, 0.01382443382099928647, 0.01481152611431567345, 0.01579861840763206043 ),
 .UNSPECIFIED. ) ;
#11660=CARTESIAN_POINT ( 'NONE',  ( -4.695048959678141287, 66.33121464499512854, 5.333703082175816235 ) ) ;
#11665=DIRECTION ( 'NONE',  ( 0.000000000000000000, 0.000000000000000000, -1.000000000000000000 ) ) ;
#11667=CYLINDRICAL_SURFACE ( 'NONE', #8917, 15.00000000000000000 ) ;
#11679=DIRECTION ( 'NONE',  ( 0.000000000000000000, 1.000000000000000000, 0.000000000000000000 ) ) ;
#11693=CARTESIAN_POINT ( 'NONE',  ( -22.75605871197916130, 79.99999999991582911, -10.56315151873249647 ) ) ;
#11698=DIRECTION ( 'NONE',  ( 0.000000000000000000, -1.000000000000000000, 0.000000000000000000 ) ) ;
#11703=EDGE_LOOP ( 'NONE', ( #18717, #13993, #6325, #18530 ) ) ;
#11707=CARTESIAN_POINT ( 'NONE',  ( -2.548407363833455452, 77.71408077849609697, -4.406821185032912425 ) ) ;
#11715=CARTESIAN_POINT ( 'NONE',  ( -30.96704536876718095, 79.01393351695151068, -7.140257836325814012 ) ) ;
#11717=CARTESIAN_POINT ( 'NONE',  ( -28.48198157863886948, 6.472551248386185563, 0.7817513343805246873 ) ) ;
#11726=CARTESIAN_POINT ( 'NONE',  ( 27.66668267600675435, 64.25000000000000000, 1.813692929321166547 ) ) ;
#11727=CARTESIAN_POINT ( 'NONE',  ( -3.504048379385980017, 53.26946170535641301, -3.147386235863720128 ) ) ;
#11728=CARTESIAN_POINT ( 'NONE',  ( 1.439239224086409141, 76.85170763124995119, -3.302610618814554311 ) ) ;
#11738=DIRECTION ( 'NONE',  ( -1.000000000000000000, -0.000000000000000000, -0.000000000000000000 ) ) ;
#11741=ORIENTED_EDGE ( 'NONE', *, *, #17815, .F. ) ;
#11752=CARTESIAN_POINT ( 'NONE',  ( -15.99999999999999289, 15.09941697557068530, 15.00000000000000000 ) ) ;
#11753=CARTESIAN_POINT ( 'NONE',  ( -33.12132922318642869, 51.54497531638352115, -5.859852249581638972 ) ) ;
#11773=CIRCLE ( 'NONE', #5669, 13.99999999999998757 ) ;
#11778=CARTESIAN_POINT ( 'NONE',  ( -15.99999999999999289, 9.999999999999994671, 0.000000000000000000 ) ) ;
#11779=DIRECTION ( 'NONE',  ( -0.000000000000000000, -1.000000000000000000, -0.000000000000000000 ) ) ;
#11783=DIRECTION ( 'NONE',  ( -0.000000000000000000, 1.000000000000000000, -0.000000000000000000 ) ) ;
#11788=CARTESIAN_POINT ( 'NONE',  ( -11.79233082830550217, 67.16614382405823847, -2.712160011935105697 ) ) ;
#11793=ORIENTED_EDGE ( 'NONE', *, *, #3004, .F. ) ;
#11795=VERTEX_POINT ( 'NONE', #9774 ) ;
#11797=CARTESIAN_POINT ( 'NONE',  ( -22.93365594915012906, 79.93797039651411751, -11.02074839552765440 ) ) ;
#11810=CARTESIAN_POINT ( 'NONE',  ( -10.36721944571354292, 79.98685641808548041, -11.85964839586857700 ) ) ;
#11812=VERTEX_POINT ( 'NONE', #7880 ) ;
#11814=DIRECTION ( 'NONE',  ( 0.000000000000000000, 0.000000000000000000, -1.000000000000000000 ) ) ;
#11819=CARTESIAN_POINT ( 'NONE',  ( -27.12336767588134379, 6.223326257262052685, 5.765760347548625653 ) ) ;
#11825=EDGE_CURVE ( 'NONE', #9665, #9995, #20725, .T. ) ;
#11830=CARTESIAN_POINT ( 'NONE',  ( 0.2566486213402327521, 60.25789211473291118, 1.735236065182640397 ) ) ;
#11831=CARTESIAN_POINT ( 'NONE',  ( -15.99999999999999289, 80.00000000000000000, -12.50000000000000000 ) ) ;
#11839=LINE ( 'NONE', #8957, #1050 ) ;
#11841=ORIENTED_EDGE ( 'NONE', *, *, #15924, .F. ) ;
#11857=DIRECTION ( 'NONE',  ( 0.000000000000000000, 0.000000000000000000, -1.000000000000000000 ) ) ;
#11858=CARTESIAN_POINT ( 'NONE',  ( -26.63192765507035276, 50.95949204697693347, -6.673528889801894515 ) ) ;
#11867=CIRCLE ( 'NONE', #8457, 12.50000000000000000 ) ;
#11868=ORIENTED_EDGE ( 'NONE', *, *, #11344, .F. ) ;
#11869=EDGE_CURVE ( 'NONE', #14773, #15680, #17349, .T. ) ;
#11871=FACE_BOUND ( 'NONE', #2062, .T. ) ;
#11877=EDGE_CURVE ( 'NONE', #20090, #3073, #1770, .T. ) ;
#11899=DIRECTION ( 'NONE',  ( 0.000000000000000000, -1.000000000000000000, 0.000000000000000000 ) ) ;
#11903=AXIS2_PLACEMENT_3D ( 'NONE', #17339, #9258, #1225 ) ;
#11907=CARTESIAN_POINT ( 'NONE',  ( -18.07003674992471431, 79.99999999999891998, -12.33825502280018860 ) ) ;
#11911=AXIS2_PLACEMENT_3D ( 'NONE', #12790, #11397, #15868 ) ;
#11913=AXIS2_PLACEMENT_3D ( 'NONE', #1054, #17265, #4334 ) ;
#11920=LINE ( 'NONE', #17002, #9818 ) ;
#11922=CARTESIAN_POINT ( 'NONE',  ( -2.776596111954927171, 78.20541348178335284, -5.222231676844829806 ) ) ;
#11926=LINE ( 'NONE', #8627, #4114 ) ;
#11932=EDGE_CURVE ( 'NONE', #16360, #13235, #8509, .T. ) ;
#11933=CARTESIAN_POINT ( 'NONE',  ( -26.20390737937308501, 9.999999997134366936, 7.228123494169216734 ) ) ;
#11941=CARTESIAN_POINT ( 'NONE',  ( -3.331652052620986737, 63.24197008610744319, 2.417743185958345364 ) ) ;
#11952=DIRECTION ( 'NONE',  ( 1.000000000000000000, 0.000000000000000000, 0.000000000000000000 ) ) ;
#11954=ORIENTED_EDGE ( 'NONE', *, *, #9087, .F. ) ;
#11962=CARTESIAN_POINT ( 'NONE',  ( -20.18890516563201487, 67.16713051729674078, -2.731108915583016383 ) ) ;
#11967=CARTESIAN_POINT ( 'NONE',  ( -26.07892689538028819, 45.11091634825275776, -7.401594269996666142 ) ) ;
#11969=B_SPLINE_CURVE_WITH_KNOTS ( 'NONE', 3,
 ( #1488, #2082, #11726, #19769 ),
 .UNSPECIFIED., .F., .F.,
 ( 4, 4 ),
 ( 0.000000000000000000, 0.001415162808320492545 ),
 .UNSPECIFIED. ) ;
#11977=VERTEX_POINT ( 'NONE', #13612 ) ;
#11980=DIRECTION ( 'NONE',  ( 0.000000000000000000, -0.000000000000000000, -1.000000000000000000 ) ) ;
#12002=VERTEX_POINT ( 'NONE', #13394 ) ;
#12003=DIRECTION ( 'NONE',  ( 0.000000000000000000, 1.000000000000000000, -0.000000000000000000 ) ) ;
#12006=EDGE_LOOP ( 'NONE', ( #15485, #7043, #4954, #5855 ) ) ;
#12011=CARTESIAN_POINT ( 'NONE',  ( -17.04272031725003700, 79.99998834348832588, -12.47960036978351539 ) ) ;
#12025=CARTESIAN_POINT ( 'NONE',  ( -14.69781867356227245, 79.99997331865614569, -12.46740305798945592 ) ) ;
#12036=CARTESIAN_POINT ( 'NONE',  ( -28.14271859785574748, 6.485482021666785890, 3.095587321074997789 ) ) ;
#12037=CARTESIAN_POINT ( 'NONE',  ( -15.99999999999999289, 80.00000000000000000, -4.999999999999989342 ) ) ;
#12043=DIRECTION ( 'NONE',  ( 0.000000000000000000, 1.000000000000000000, 0.000000000000000000 ) ) ;
#12060=DIRECTION ( 'NONE',  ( 0.000000000000000000, -1.000000000000000000, 0.000000000000000000 ) ) ;
#12067=CARTESIAN_POINT ( 'NONE',  ( -14.28506451248627940, 45.59460031122257107, -12.38656090347159022 ) ) ;
#12072=EDGE_CURVE ( 'NONE', #5803, #15680, #7542, .T. ) ;
#12073=EDGE_LOOP ( 'NONE', ( #5848, #2847 ) ) ;
#12078=AXIS2_PLACEMENT_3D ( 'NONE', #7267, #2203, #5252 ) ;
#12081=EDGE_LOOP ( 'NONE', ( #13624, #11061, #16911, #5012 ) ) ;
#12082=ORIENTED_EDGE ( 'NONE', *, *, #11156, .F. ) ;
#12087=CARTESIAN_POINT ( 'NONE',  ( -13.48328391324397657, 19.43205798116640537, 12.24715376271861800 ) ) ;
#12088=AXIS2_PLACEMENT_3D ( 'NONE', #3967, #13518, #7138 ) ;
#12094=CARTESIAN_POINT ( 'NONE',  ( -28.02004479723489894, 75.03053098945940746, 3.432994178266289165 ) ) ;
#12099=CARTESIAN_POINT ( 'NONE',  ( -3.768439905627497755, 65.75000000000002842, 3.993547312438780583 ) ) ;
#12109=ORIENTED_EDGE ( 'NONE', *, *, #20343, .F. ) ;
#12118=DIRECTION ( 'NONE',  ( -0.000000000000000000, 1.000000000000000000, -0.000000000000000000 ) ) ;
#12124=CARTESIAN_POINT ( 'NONE',  ( 10.49211908931699178, -24.14213562373095456, -5.000000000000000000 ) ) ;
#12129=ORIENTED_EDGE ( 'NONE', *, *, #10561, .T. ) ;
#12132=CARTESIAN_POINT ( 'NONE',  ( 28.00000000000001066, 64.25000000000000000, 1.479896280015810639 ) ) ;
#12133=ORIENTED_EDGE ( 'NONE', *, *, #422, .T. ) ;
#12137=CARTESIAN_POINT ( 'NONE',  ( -27.65088713606887438, 9.446972530103739274, 4.576488380515961296 ) ) ;
#12161=CARTESIAN_POINT ( 'NONE',  ( 30.10683012259193703, -10.00000000000000000, 0.000000000000000000 ) ) ;
#12165=CARTESIAN_POINT ( 'NONE',  ( -17.40260810207333719, 71.39595272406131699, -4.812026853405401816 ) ) ;
#12167=AXIS2_PLACEMENT_3D ( 'NONE', #7072, #8561, #15059 ) ;
#12171=CARTESIAN_POINT ( 'NONE',  ( -23.40647577390874545, 45.06233805004389836, -10.07534141557004226 ) ) ;
#12181=AXIS2_PLACEMENT_3D ( 'NONE', #19356, #4418, #8001 ) ;
#12184=CARTESIAN_POINT ( 'NONE',  ( 10.49211908931699178, 0.000000000000000000, 5.999999999999998224 ) ) ;
#12194=CARTESIAN_POINT ( 'NONE',  ( -11.51383524490820420, 17.33161812738734753, 11.66803293973013389 ) ) ;
#12195=( BOUNDED_CURVE ( )  B_SPLINE_CURVE ( 3, ( #6237, #20458, #5925, #17183 ),
 .UNSPECIFIED., .F., .F. ) 
 B_SPLINE_CURVE_WITH_KNOTS ( ( 4, 4 ),
 ( 3.141592653589793116, 4.511031059594355241 ),
 .UNSPECIFIED. ) 
 CURVE ( )  GEOMETRIC_REPRESENTATION_ITEM ( )  RATIONAL_B_SPLINE_CURVE ( ( 1.000000000000000000, 0.8497311128276563430, 0.8497311128276563430, 1.000000000000000000 ) ) 
 REPRESENTATION_ITEM ( '' )  );
#12202=CARTESIAN_POINT ( 'NONE',  ( -28.45830647201975694, 79.08610913873366144, 1.260722419664553673 ) ) ;
#12216=CIRCLE ( 'NONE', #8830, 4.999999999999995559 ) ;
#12222=LINE ( 'NONE', #4266, #14407 ) ;
#12232=CARTESIAN_POINT ( 'NONE',  ( 0.000000000000000000, 5.000000000000000000, -30.00000000000000000 ) ) ;
#12236=CARTESIAN_POINT ( 'NONE',  ( -20.40277896402405133, 18.53029315133363752, 3.430876175762952673 ) ) ;
#12254=AXIS2_PLACEMENT_3D ( 'NONE', #5499, #5391, #20037 ) ;
#12256=AXIS2_PLACEMENT_3D ( 'NONE', #6075, #9359, #17756 ) ;
#12258=EDGE_LOOP ( 'NONE', ( #15333, #12133, #347, #14898, #8698, #6017, #5979 ) ) ;
#12267=CARTESIAN_POINT ( 'NONE',  ( 26.99999999999999645, 64.25000000000000000, -2.528164662410438357 ) ) ;
#12268=AXIS2_PLACEMENT_3D ( 'NONE', #19741, #5209, #3949 ) ;
#12270=AXIS2_PLACEMENT_3D ( 'NONE', #16731, #8562, #11857 ) ;
#12277=EDGE_CURVE ( 'NONE', #4912, #9631, #17624, .T. ) ;
#12288=CARTESIAN_POINT ( 'NONE',  ( -15.31857793801784062, 45.63007274853293893, -12.48623160004378363 ) ) ;
#12292=ORIENTED_EDGE ( 'NONE', *, *, #618, .F. ) ;
#12300=EDGE_LOOP ( 'NONE', ( #12129, #13699, #6981, #12325, #14373, #9678 ) ) ;
#12302=FACE_OUTER_BOUND ( 'NONE', #6186, .T. ) ;
#12303=CARTESIAN_POINT ( 'NONE',  ( 0.8775796894216562061, 57.25228208760839266, 0.3499516663593752464 ) ) ;
#12312=PLANE ( 'NONE',  #8931 ) ;
#12322=DIRECTION ( 'NONE',  ( 0.000000000000000000, 0.000000000000000000, -1.000000000000000000 ) ) ;
#12323=ORIENTED_EDGE ( 'NONE', *, *, #17421, .T. ) ;
#12325=ORIENTED_EDGE ( 'NONE', *, *, #8214, .F. ) ;
#12341=B_SPLINE_CURVE_WITH_KNOTS ( 'NONE', 3,
 ( #8135, #3273, #7729, #1688, #13039, #19478, #2870, #9306, #1282, #12624, #6134, #14852, #2002, #10028, #13244, #3583, #3792, #5367, #13138, #15168, #16523, #5265 ),
 .UNSPECIFIED., .F., .F.,
 ( 4, 2, 2, 2, 2, 2, 2, 2, 2, 2, 4 ),
 ( 0.01579861840763206043, 0.01629201531149390356, 0.01678541221535574668, 0.01777220602307943639, 0.01875899983080312264, 0.01974579363852681235, 0.02073258744625049860, 0.02122598435011234519, 0.02171938125397419178, 0.02270617506169788843, 0.02369296886942158509 ),
 .UNSPECIFIED. ) ;
#12354=ORIENTED_EDGE ( 'NONE', *, *, #18046, .T. ) ;
#12368=DIRECTION ( 'NONE',  ( 0.000000000000000000, 0.000000000000000000, -1.000000000000000000 ) ) ;
#12391=CARTESIAN_POINT ( 'NONE',  ( -21.34090909479325759, 45.27736777337857887, -11.32243216392325458 ) ) ;
#12405=CARTESIAN_POINT ( 'NONE',  ( -33.21445101426393620, 51.72190322358105874, -5.511193331917786153 ) ) ;
#12428=AXIS2_PLACEMENT_3D ( 'NONE', #9058, #13644, #12368 ) ;
#12429=EDGE_CURVE ( 'NONE', #13646, #5066, #5287, .T. ) ;
#12434=CARTESIAN_POINT ( 'NONE',  ( -4.015193415984987801, 74.73312780907788522, 3.553696893467043871 ) ) ;
#12449=CARTESIAN_POINT ( 'NONE',  ( -4.442041072745785080, 70.83821676753269969, 4.766221741044108562 ) ) ;
#12469=FACE_OUTER_BOUND ( 'NONE', #16330, .T. ) ;
#12471=ORIENTED_EDGE ( 'NONE', *, *, #15754, .T. ) ;
#12477=CARTESIAN_POINT ( 'NONE',  ( -18.23302563531977327, 10.61358200216139203, 12.30279443686337082 ) ) ;
#12482=DIRECTION ( 'NONE',  ( -0.000000000000000000, -1.000000000000000000, 0.000000000000000000 ) ) ;
#12483=EDGE_CURVE ( 'NONE', #13646, #6959, #12963, .T. ) ;
#12488=CARTESIAN_POINT ( 'NONE',  ( -22.50947703420033008, 49.61991195516749542, -10.68093576282688240 ) ) ;
#12492=EDGE_LOOP ( 'NONE', ( #2672, #7528, #15241, #8012, #12760 ) ) ;
#12496=CARTESIAN_POINT ( 'NONE',  ( -3.580465574138951723, 80.00000000005285017, -1.424835221694952025 ) ) ;
#12501=CARTESIAN_POINT ( 'NONE',  ( -33.51494856915631715, 53.43435578398468522, -2.915686290500575151 ) ) ;
#12502=CARTESIAN_POINT ( 'NONE',  ( -26.77504448057880637, 9.902224835466700625, 6.371987388190586188 ) ) ;
#12511=CARTESIAN_POINT ( 'NONE',  ( 28.00000000000001066, 64.25000000000000000, 75.00000000000000000 ) ) ;
#12516=CARTESIAN_POINT ( 'NONE',  ( -28.45531017328980994, 78.99734867018936768, 1.332611642696158505 ) ) ;
#12519=FACE_OUTER_BOUND ( 'NONE', #11185, .T. ) ;
#12522=EDGE_CURVE ( 'NONE', #10554, #6749, #13982, .T. ) ;
#12524=ORIENTED_EDGE ( 'NONE', *, *, #19194, .T. ) ;
#12528=CARTESIAN_POINT ( 'NONE',  ( -3.057294037196384817, 74.04855861174505094, -0.5148205403777549316 ) ) ;
#12534=ADVANCED_FACE ( 'NONE', ( #20555 ), #15600, .T. ) ;
#12546=CARTESIAN_POINT ( 'NONE',  ( -15.99999999999999289, 20.09941697557067997, 4.999999999999989342 ) ) ;
#12569=DIRECTION ( 'NONE',  ( -0.000000000000000000, -1.000000000000000000, -0.000000000000000000 ) ) ;
#12583=CARTESIAN_POINT ( 'NONE',  ( -16.33019277271582226, 10.09941697557068707, 12.50000000000000178 ) ) ;
#12584=LINE ( 'NONE', #17354, #13256 ) ;
#12592=MECHANICAL_DESIGN_GEOMETRIC_PRESENTATION_REPRESENTATION('',(#6820),#15663);
#12594=CARTESIAN_POINT ( 'NONE',  ( -8.885764546551122578, 45.08372817709340552, -10.30101951839246333 ) ) ;
#12605=CARTESIAN_POINT ( 'NONE',  ( -3.645413219200714039, 80.00000000007608492, -1.908121642414585484 ) ) ;
#12607=VERTEX_POINT ( 'NONE', #4141 ) ;
#12611=CARTESIAN_POINT ( 'NONE',  ( -16.80570248528584543, 50.47613221401184802, -16.24930194057697364 ) ) ;
#12612=CARTESIAN_POINT ( 'NONE',  ( -27.37786364650417070, 9.617207265011291639, -5.186836524664776071 ) ) ;
#12623=CARTESIAN_POINT ( 'NONE',  ( -27.89556006008164246, 56.02656468610143037, 3.843087363396194611 ) ) ;
#12624=CARTESIAN_POINT ( 'NONE',  ( -19.97143893519406888, 18.15431163985882890, 11.85386933495461825 ) ) ;
#12625=EDGE_LOOP ( 'NONE', ( #20594, #11240, #10902 ) ) ;
#12637=CARTESIAN_POINT ( 'NONE',  ( -3.633681703949028119, 78.08772077735648054, 1.916778294983234154 ) ) ;
#12639=CARTESIAN_POINT ( 'NONE',  ( -16.47102837334524850, 80.00000000000002842, -12.49810385314669148 ) ) ;
#12644=CARTESIAN_POINT ( 'NONE',  ( 27.00000000000002487, 64.25000000000000000, 2.481238266578627449 ) ) ;
#12648=CARTESIAN_POINT ( 'NONE',  ( 0.2286262486868663735, 60.41611051155134504, 1.787729794976060660 ) ) ;
#12649=DIRECTION ( 'NONE',  ( -1.000000000000000000, 0.000000000000000000, 0.000000000000000000 ) ) ;
#12651=EDGE_CURVE ( 'NONE', #17792, #4687, #9521, .T. ) ;
#12654=FACE_OUTER_BOUND ( 'NONE', #15335, .T. ) ;
#12656=CYLINDRICAL_SURFACE ( 'NONE', #3720, 13.99999999999999822 ) ;
#12659=CARTESIAN_POINT ( 'NONE',  ( -20.99999999999998224, 15.09941697557068530, 15.00000000000000000 ) ) ;
#12662=CARTESIAN_POINT ( 'NONE',  ( -28.50352467013047431, 79.99999999992598987, -0.04629550956175955412 ) ) ;
#12681=CARTESIAN_POINT ( 'NONE',  ( -14.99999999999999645, 0.000000000000000000, -28.99999999999999645 ) ) ;
#12689=CARTESIAN_POINT ( 'NONE',  ( -19.97299960082356307, 12.04641549374639276, 11.85335538211749018 ) ) ;
#12698=CARTESIAN_POINT ( 'NONE',  ( -7.715557909791129987, 49.87593469365641141, -9.365636588568600374 ) ) ;
#12706=DIRECTION ( 'NONE',  ( -1.000000000000000000, -0.000000000000000000, -0.000000000000000000 ) ) ;
#12710=DIRECTION ( 'NONE',  ( -0.000000000000000000, 1.000000000000000000, -0.000000000000000000 ) ) ;
#12713=CARTESIAN_POINT ( 'NONE',  ( -28.38583607363177208, 8.722028531692911812, -1.718349999867211597 ) ) ;
#12719=EDGE_CURVE ( 'NONE', #4703, #681, #19287, .T. ) ;
#12721=CARTESIAN_POINT ( 'NONE',  ( -27.32538345582499772, 67.03307707865299392, 5.290582662559629945 ) ) ;
#12732=CARTESIAN_POINT ( 'NONE',  ( -3.601598805479791388, 64.25000000000000000, 3.829763509598321125 ) ) ;
#12734=EDGE_CURVE ( 'NONE', #245, #10584, #12341, .T. ) ;
#12735=CARTESIAN_POINT ( 'NONE',  ( -17.86792573809073303, 79.99987962855902879, -12.43445577838060245 ) ) ;
#12739=CARTESIAN_POINT ( 'NONE',  ( 10.49211908931699178, -10.00000000000000000, 0.000000000000000000 ) ) ;
#12743=CARTESIAN_POINT ( 'NONE',  ( -0.08752631476754749174, 62.68128730906327917, 2.340095601044604567 ) ) ;
#12750=CIRCLE ( 'NONE', #7312, 5.000000000000000000 ) ;
#12753=CARTESIAN_POINT ( 'NONE',  ( -13.51899739228861463, 20.09941697557067641, 4.999999999999990230 ) ) ;
#12759=CARTESIAN_POINT ( 'NONE',  ( -20.89897948556633978, 16.09941697557071905, 0.9999999999999991118 ) ) ;
#12760=ORIENTED_EDGE ( 'NONE', *, *, #10117, .T. ) ;
#12764=DIRECTION ( 'NONE',  ( 1.000000000000000000, 0.000000000000000000, 0.000000000000000000 ) ) ;
#12771=CARTESIAN_POINT ( 'NONE',  ( -26.96929348833892703, 80.00000000026912517, -6.044438231901797742 ) ) ;
#12790=CARTESIAN_POINT ( 'NONE',  ( -15.99999999999999289, 9.999999999999994671, 0.000000000000000000 ) ) ;
#12801=CARTESIAN_POINT ( 'NONE',  ( -4.278641067966838740, 51.99310020370139540, -4.954688218471713590 ) ) ;
#12807=AXIS2_PLACEMENT_3D ( 'NONE', #20368, #10937, #9224 ) ;
#12812=DIRECTION ( 'NONE',  ( 0.000000000000000000, -1.000000000000000000, 0.000000000000000000 ) ) ;
#12814=CARTESIAN_POINT ( 'NONE',  ( -4.127064941938266784, 79.99999999978183496, -3.927153389735459132 ) ) ;
#12819=CARTESIAN_POINT ( 'NONE',  ( -20.28206330180632833, 63.53129375914073762, -2.582219875156735345 ) ) ;
#12822=CARTESIAN_POINT ( 'NONE',  ( -28.39001627391951388, 8.716765542848399662, 1.688643308777810992 ) ) ;
#12829=CARTESIAN_POINT ( 'NONE',  ( -29.99999999999999645, 5.000000000000000000, 15.00000000000000000 ) ) ;
#12830=CARTESIAN_POINT ( 'NONE',  ( -27.38197634705172234, 68.30950415664236175, 5.167706431871533113 ) ) ;
#12835=ORIENTED_EDGE ( 'NONE', *, *, #6255, .T. ) ;
#12844=B_SPLINE_CURVE_WITH_KNOTS ( 'NONE', 3,
 ( #9112, #15614, #6998, #11136, #12732, #1494, #4360, #7941, #2778, #16032, #9219, #6344, #14443, #5932 ),
 .UNSPECIFIED., .F., .F.,
 ( 4, 2, 2, 2, 2, 2, 4 ),
 ( 0.000000000000000000, 0.001404861450950275039, 0.002107292176425411365, 0.002809722901900548343, 0.003512153627375684886, 0.004214584352850820996, 0.005619445803801094083 ),
 .UNSPECIFIED. ) ;
#12849=APPLICATION_CONTEXT ( 'automotive_design' ) ;
#12850=PLANE ( 'NONE',  #20265 ) ;
#12853=VECTOR ( 'NONE', #19813, 1000.000000000000000 ) ;
#12863=DIRECTION ( 'NONE',  ( 0.000000000000000000, 0.000000000000000000, -1.000000000000000000 ) ) ;
#12869=DIRECTION ( 'NONE',  ( 0.000000000000000000, 0.000000000000000000, 1.000000000000000000 ) ) ;
#12871=AXIS2_PLACEMENT_3D ( 'NONE', #14619, #16295, #1561 ) ;
#12875=CARTESIAN_POINT ( 'NONE',  ( -28.46762626707359445, 79.99999999989459809, -0.9530258780664238039 ) ) ;
#12881=DIRECTION ( 'NONE',  ( -0.000000000000000000, -1.000000000000000000, -0.000000000000000000 ) ) ;
#12887=ORIENTED_EDGE ( 'NONE', *, *, #15373, .F. ) ;
#12888=DIRECTION ( 'NONE',  ( 0.000000000000000000, 0.000000000000000000, -1.000000000000000000 ) ) ;
#12898=CARTESIAN_POINT ( 'NONE',  ( -29.99999999999963052, 5.000000000000220268, -4.654981692112267311 ) ) ;
#12900=EDGE_LOOP ( 'NONE', ( #8357, #16863, #19396, #20584, #10784, #10675, #4007, #16738, #3052, #7348, #8177, #14608 ) ) ;
#12906=CARTESIAN_POINT ( 'NONE',  ( -0.8702360668455834114, 50.25436005864763445, -9.730529323853312818 ) ) ;
#12907=DIRECTION ( 'NONE',  ( 0.000000000000000000, 0.000000000000000000, -1.000000000000000000 ) ) ;
#12912=VERTEX_POINT ( 'NONE', #13664 ) ;
#12918=CARTESIAN_POINT ( 'NONE',  ( -2.526178703648428669, 77.46132694877630342, -4.041171758127903857 ) ) ;
#12922=CARTESIAN_POINT ( 'NONE',  ( -19.54621117075676651, 60.56420712653811478, -3.531915534904321419 ) ) ;
#12926=ORIENTED_EDGE ( 'NONE', *, *, #17508, .T. ) ;
#12934=CIRCLE ( 'NONE', #19351, 11.00000000000001066 ) ;
#12936=FACE_OUTER_BOUND ( 'NONE', #19926, .T. ) ;
#12963=CIRCLE ( 'NONE', #11590, 5.999999999999998224 ) ;
#12969=ORIENTED_EDGE ( 'NONE', *, *, #6831, .F. ) ;
#12979=CIRCLE ( 'NONE', #3818, 9.999999999999998224 ) ;
#12983=CARTESIAN_POINT ( 'NONE',  ( -28.78765050820362603, 78.65050410969298866, -6.103909342518194059 ) ) ;
#12985=CARTESIAN_POINT ( 'NONE',  ( -15.99999999999999289, 64.25000000000000000, 0.000000000000000000 ) ) ;
#12988=CARTESIAN_POINT ( 'NONE',  ( -29.98143750865132162, 64.25000000000000000, 2.826871295670245310 ) ) ;
#12997=DIRECTION ( 'NONE',  ( 0.000000000000000000, 0.000000000000000000, -1.000000000000000000 ) ) ;
#13010=EDGE_CURVE ( 'NONE', #4238, #16527, #12979, .T. ) ;
#13012=CARTESIAN_POINT ( 'NONE',  ( -11.30699436262336022, 45.34934999665991029, -11.59074373136150271 ) ) ;
#13015=CARTESIAN_POINT ( 'NONE',  ( -19.79889058375756861, 45.44132677019771904, -11.91506545529773753 ) ) ;
#13020=CARTESIAN_POINT ( 'NONE',  ( -20.40277896402405133, 11.66854079980773307, 3.430876175762952673 ) ) ;
#13033=EDGE_CURVE ( 'NONE', #6749, #13669, #6509, .T. ) ;
#13038=CARTESIAN_POINT ( 'NONE',  ( -28.04417108971878037, 54.76469415528241313, 3.349407265930378408 ) ) ;
#13039=CARTESIAN_POINT ( 'NONE',  ( -20.93440336536924562, 15.92340406867066882, 11.48489954023713899 ) ) ;
#13048=EDGE_LOOP ( 'NONE', ( #7934, #8327, #14099, #16372 ) ) ;
#13056=ORIENTED_EDGE ( 'NONE', *, *, #3301, .T. ) ;
#13073=CARTESIAN_POINT ( 'NONE',  ( -15.11015962792897227, 71.52657754998247697, -4.923257761629217910 ) ) ;
#13085=CARTESIAN_POINT ( 'NONE',  ( -28.23783794168646466, 80.00000000009136158, -2.568690455535888262 ) ) ;
#13098=DIRECTION ( 'NONE',  ( 0.000000000000000000, -1.000000000000000000, 0.000000000000000000 ) ) ;
#13101=CYLINDRICAL_SURFACE ( 'NONE', #7139, 12.50000000000000000 ) ;
#13108=AXIS2_PLACEMENT_3D ( 'NONE', #7931, #5923, #9523 ) ;
#13109=CARTESIAN_POINT ( 'NONE',  ( -15.22417136430887119, 45.62850095463065259, -12.48193588431748324 ) ) ;
#13111=CARTESIAN_POINT ( 'NONE',  ( -0.01127596767515291407, 61.98808745880752724, 2.211961002137901922 ) ) ;
#13112=DIRECTION ( 'NONE',  ( -0.000000000000000000, -1.000000000000000000, -0.000000000000000000 ) ) ;
#13121=ORIENTED_EDGE ( 'NONE', *, *, #13190, .T. ) ;
#13123=CARTESIAN_POINT ( 'NONE',  ( -17.39810202520303406, 58.61478893848392602, -4.803508630518933842 ) ) ;
#13137=CARTESIAN_POINT ( 'NONE',  ( -28.81347165278748790, 54.47717305474855465, -1.798637628744577555 ) ) ;
#13138=CARTESIAN_POINT ( 'NONE',  ( -17.30956942029561674, 19.93606970371389764, 12.43541898840899940 ) ) ;
#13141=CARTESIAN_POINT ( 'NONE',  ( -15.99999999999999289, 0.000000000000000000, 5.999999999999989342 ) ) ;
#13155=CARTESIAN_POINT ( 'NONE',  ( -30.20082347186430027, 65.74999999999995737, 2.745993778453658773 ) ) ;
#13164=LINE ( 'NONE', #9851, #3732 ) ;
#13167=CIRCLE ( 'NONE', #6704, 5.999999999999989342 ) ;
#13170=EDGE_CURVE ( 'NONE', #8072, #2271, #10770, .T. ) ;
#13185=CARTESIAN_POINT ( 'NONE',  ( -28.35458678079950445, 80.00000000007563017, -1.908121642414536856 ) ) ;
#13189=VERTEX_POINT ( 'NONE', #274 ) ;
#13190=EDGE_CURVE ( 'NONE', #9995, #10584, #1769, .T. ) ;
#13194=CARTESIAN_POINT ( 'NONE',  ( -28.95046476526206192, 64.25000000000000000, 3.381771649840967342 ) ) ;
#13207=CARTESIAN_POINT ( 'NONE',  ( -15.00000000000000000, 0.000000000000000000, 28.99999999999999645 ) ) ;
#13209=CARTESIAN_POINT ( 'NONE',  ( -28.99999999999999289, 0.000000000000000000, 15.00000000000000178 ) ) ;
#13214=CARTESIAN_POINT ( 'NONE',  ( -3.815209910797584314, 53.56373870034735063, 2.796190595711027793 ) ) ;
#13219=EDGE_CURVE ( 'NONE', #6749, #7840, #11288, .T. ) ;
#13229=ORIENTED_EDGE ( 'NONE', *, *, #11349, .T. ) ;
#13233=CARTESIAN_POINT ( 'NONE',  ( -12.32033641378040834, 60.86279337894578134, -3.389612121674974610 ) ) ;
#13235=VERTEX_POINT ( 'NONE', #18903 ) ;
#13243=CARTESIAN_POINT ( 'NONE',  ( -33.34256115809776588, 52.05794329512087160, -4.908380826879679582 ) ) ;
#13244=CARTESIAN_POINT ( 'NONE',  ( -18.51262115207460823, 19.42532919514705370, 12.24574540514312204 ) ) ;
#13247=DIRECTION ( 'NONE',  ( 0.000000000000000000, 0.000000000000000000, -1.000000000000000000 ) ) ;
#13254=CARTESIAN_POINT ( 'NONE',  ( -3.332456710801453337, 66.65723886914538809, 2.419320319694736376 ) ) ;
#13256=VECTOR ( 'NONE', #6088, 1000.000000000000000 ) ;
#13261=CARTESIAN_POINT ( 'NONE',  ( -31.82323003959540486, 65.74999999999997158, 2.481238266578629226 ) ) ;
#13262=ORIENTED_EDGE ( 'NONE', *, *, #6924, .F. ) ;
#13273=EDGE_CURVE ( 'NONE', #3253, #20919, #17728, .T. ) ;
#13278=CARTESIAN_POINT ( 'NONE',  ( -12.32004792737159882, 69.13648218375620047, -3.389291572743964753 ) ) ;
#13288=CARTESIAN_POINT ( 'NONE',  ( -16.52214153618450254, 80.00000165566777355, -12.49590370130044903 ) ) ;
#13290=CARTESIAN_POINT ( 'NONE',  ( -15.00000000000000000, -10.00000000000000000, 28.99999999999999645 ) ) ;
#13304=CARTESIAN_POINT ( 'NONE',  ( -13.92996325007571379, 79.99999999999890576, -12.33825502280066111 ) ) ;
#13310=DIRECTION ( 'NONE',  ( 0.000000000000000000, 0.000000000000000000, -1.000000000000000000 ) ) ;
#13314=CARTESIAN_POINT ( 'NONE',  ( -30.00000000000040146, 4.999999999999647393, -3.756581053969355821 ) ) ;
#13323=CARTESIAN_POINT ( 'NONE',  ( 1.287529140580364606, 55.27775868348017241, -1.071617489983800908 ) ) ;
#13324=CARTESIAN_POINT ( 'NONE',  ( -0.1082929358729399077, 78.60836521392512566, -6.178814694513294015 ) ) ;
#13337=DIRECTION ( 'NONE',  ( 0.000000000000000000, 0.000000000000000000, -1.000000000000000000 ) ) ;
#13341=DIRECTION ( 'NONE',  ( 0.000000000000000000, -1.000000000000000000, 0.000000000000000000 ) ) ;
#13348=CARTESIAN_POINT ( 'NONE',  ( -28.43641358195718283, 53.09495409546831013, -3.357527245236496594 ) ) ;
#13389=CIRCLE ( 'NONE', #14772, 4.999999999999990230 ) ;
#13391=CARTESIAN_POINT ( 'NONE',  ( -15.00000000000000000, 0.000000000000000000, 28.99999999999999645 ) ) ;
#13394=CARTESIAN_POINT ( 'NONE',  ( -15.99999999999999289, 64.25000000000000000, 4.999999999999989342 ) ) ;
#13404=CARTESIAN_POINT ( 'NONE',  ( -3.762162058313276436, 80.00000000009157475, -2.568690455533788164 ) ) ;
#13411=CARTESIAN_POINT ( 'NONE',  ( -31.89200696759080600, 78.60820088387509941, -6.178462522043184357 ) ) ;
#13421=CARTESIAN_POINT ( 'NONE',  ( -3.502006981982628719, 48.75774031421161681, -0.5664283305349653297 ) ) ;
#13426=CARTESIAN_POINT ( 'NONE',  ( -3.160111173998752854, 59.48252478531676957, 1.461028833307322694 ) ) ;
#13436=CARTESIAN_POINT ( 'NONE',  ( 27.33329038210763784, 64.25000000000000000, -2.193932927905873687 ) ) ;
#13437=CARTESIAN_POINT ( 'NONE',  ( -35.00000000000000000, 65.00000000000000000, -12.50000000000000000 ) ) ;
#13452=CARTESIAN_POINT ( 'NONE',  ( -27.70464211192128445, 45.99281090038124375, -4.438302275953727616 ) ) ;
#13467=ORIENTED_EDGE ( 'NONE', *, *, #15780, .T. ) ;
#13474=FACE_OUTER_BOUND ( 'NONE', #2328, .T. ) ;
#13479=DIRECTION ( 'NONE',  ( 0.000000000000000000, -1.000000000000000000, 0.000000000000000000 ) ) ;
#13482=CARTESIAN_POINT ( 'NONE',  ( -15.99999999999998934, 4.999999999999997335, 17.50000000000000000 ) ) ;
#13491=ORIENTED_EDGE ( 'NONE', *, *, #11471, .T. ) ;
#13492=ORIENTED_EDGE ( 'NONE', *, *, #11234, .F. ) ;
#13498=CARTESIAN_POINT ( 'NONE',  ( -18.58414241182626014, 79.99915570207093651, -12.30640999581614103 ) ) ;
#13501=ORIENTED_EDGE ( 'NONE', *, *, #9899, .T. ) ;
#13505=CARTESIAN_POINT ( 'NONE',  ( -15.99999999999999289, 9.999999999999994671, 0.000000000000000000 ) ) ;
#13512=CARTESIAN_POINT ( 'NONE',  ( -8.889222525793472940, 79.96752057144499304, -11.48167302094788589 ) ) ;
#13516=CARTESIAN_POINT ( 'NONE',  ( -15.99999999999999289, 64.25000000000000000, 0.000000000000000000 ) ) ;
#13518=DIRECTION ( 'NONE',  ( 0.000000000000000000, -1.000000000000000000, 0.000000000000000000 ) ) ;
#13529=CARTESIAN_POINT ( 'NONE',  ( -3.315871571232889448, 53.81292811603974258, -2.490183643791233692 ) ) ;
#13530=DIRECTION ( 'NONE',  ( 0.000000000000000000, 0.000000000000000000, -1.000000000000000000 ) ) ;
#13558=CARTESIAN_POINT ( 'NONE',  ( -25.95795895568129197, 50.50501676485125557, -7.579117145205284345 ) ) ;
#13573=ADVANCED_FACE ( 'NONE', ( #15090 ), #20043, .F. ) ;
#13579=CARTESIAN_POINT ( 'NONE',  ( -27.29860958162435480, 65.74999999999997158, 5.347094680480812379 ) ) ;
#13595=CIRCLE ( 'NONE', #4448, 14.99999999999999645 ) ;
#13605=ORIENTED_EDGE ( 'NONE', *, *, #17508, .F. ) ;
#13609=LINE ( 'NONE', #463, #6073 ) ;
#13612=CARTESIAN_POINT ( 'NONE',  ( 28.00000000000001066, 65.75000000000001421, 1.479896280015810639 ) ) ;
#13624=ORIENTED_EDGE ( 'NONE', *, *, #19087, .F. ) ;
#13628=CARTESIAN_POINT ( 'NONE',  ( -33.48683788045275378, 76.55850487625095013, -2.936742252775472739 ) ) ;
#13629=AXIS2_PLACEMENT_3D ( 'NONE', #8612, #11698, #10291 ) ;
#13631=CARTESIAN_POINT ( 'NONE',  ( 26.99999999999999645, 65.00000000000000000, -12.50000000000000000 ) ) ;
#13640=VECTOR ( 'NONE', #11779, 1000.000000000000000 ) ;
#13644=DIRECTION ( 'NONE',  ( 1.000000000000000000, -0.000000000000000000, -0.000000000000000000 ) ) ;
#13646=VERTEX_POINT ( 'NONE', #5189 ) ;
#13663=CARTESIAN_POINT ( 'NONE',  ( -21.23313076374843078, 50.33498419130910406, -15.65462769131217513 ) ) ;
#13664=CARTESIAN_POINT ( 'NONE',  ( -14.99999999999999645, 5.000000000000000000, -30.00000000000000000 ) ) ;
#13667=CARTESIAN_POINT ( 'NONE',  ( -27.29860958162435480, 64.25000000000000000, 5.347094680480811490 ) ) ;
#13669=VERTEX_POINT ( 'NONE', #13482 ) ;
#13675=EDGE_LOOP ( 'NONE', ( #1668, #7407, #16452, #2374, #6737, #13501, #12354, #7165, #6313 ) ) ;
#13687=AXIS2_PLACEMENT_3D ( 'NONE', #8375, #15303, #15195 ) ;
#13688=( BOUNDED_SURFACE ( )  B_SPLINE_SURFACE ( 3, 2, ( 
 ( #17611, #7637, #14133 ),
 ( #11035, #19096, #6040 ),
 ( #7530, #3084, #12637 ),
 ( #4768, #12528, #11250 ),
 ( #17719, #2880, #9317 ),
 ( #20463, #18991, #4568 ),
 ( #4470, #20669, #12434 ),
 ( #9426, #10931, #17400 ),
 ( #7740, #14239, #3184 ),
 ( #9636, #15922, #1393 ),
 ( #1081, #14021, #7841 ),
 ( #14343, #20775, #18888 ),
 ( #6243, #4666, #1598 ),
 ( #19593, #13254, #19699 ),
 ( #14658, #8143, #11660 ),
 ( #17923, #6872, #9938 ) ),
 .UNSPECIFIED., .F., .F., .F. ) 
 B_SPLINE_SURFACE_WITH_KNOTS ( ( 4, 2, 2, 2, 2, 2, 2, 4 ),
 ( 3, 3 ),
 ( 0.09394529277310079141, 0.09803747693844744315, 0.1000835690211207829, 0.1011066150624574389, 0.1021296611037941088, 0.1062218452691407744, 0.1082679373518141003, 0.1103140294344874262 ),
 ( 0.000000000000000000, 1.000000000000000000 ),
 .UNSPECIFIED. ) 
 GEOMETRIC_REPRESENTATION_ITEM ( )  RATIONAL_B_SPLINE_SURFACE ( (
 ( 1.000000000000000000, 0.7167790485004655876, 1.000000000000000000),
 ( 1.000000000000000000, 0.7312157917998172163, 1.000000000000000000),
 ( 1.000000000000000000, 0.7466500244729726843, 1.000000000000000000),
 ( 1.000000000000000000, 0.7689011243010781538, 1.000000000000000000),
 ( 1.000000000000000000, 0.7761748643737284015, 1.000000000000000000),
 ( 1.000000000000000000, 0.7866334538990542580, 1.000000000000000000),
 ( 1.000000000000000000, 0.7900487569768038787, 1.000000000000000000),
 ( 1.000000000000000000, 0.7966228133243151710, 1.000000000000000000),
 ( 1.000000000000000000, 0.7997907721098685974, 1.000000000000000000),
 ( 1.000000000000000000, 0.8149753752734353318, 1.000000000000000000),
 ( 1.000000000000000000, 0.8250225257834536974, 1.000000000000000000),
 ( 1.000000000000000000, 0.8359195949012505622, 1.000000000000000000),
 ( 1.000000000000000000, 0.8388534816486922230, 1.000000000000000000),
 ( 1.000000000000000000, 0.8430760250472538742, 1.000000000000000000),
 ( 1.000000000000000000, 0.8443918141124598931, 1.000000000000000000),
 ( 1.000000000000000000, 0.8449065510952337155, 1.000000000000000000) ) ) 
 REPRESENTATION_ITEM ( '' )  SURFACE ( )  );
#13698=CARTESIAN_POINT ( 'NONE',  ( -2.446924783487210764, 65.74999999999998579, 3.020008312198914968 ) ) ;
#13699=ORIENTED_EDGE ( 'NONE', *, *, #5004, .T. ) ;
#13700=LINE ( 'NONE', #20151, #13872 ) ;
#13701=DIRECTION ( 'NONE',  ( 6.608470384673549052E-16, -1.000000000000000000, 0.000000000000000000 ) ) ;
#13711=VERTEX_POINT ( 'NONE', #17285 ) ;
#13725=CARTESIAN_POINT ( 'NONE',  ( 10.49211908931699178, 0.000000000000000000, 0.000000000000000000 ) ) ;
#13727=ORIENTED_EDGE ( 'NONE', *, *, #616, .F. ) ;
#13732=CARTESIAN_POINT ( 'NONE',  ( -28.35621592425299653, 6.482730417836661374, 1.947608771879208556 ) ) ;
#13740=CARTESIAN_POINT ( 'NONE',  ( -34.00000000000000711, 64.25000000000000000, 2.481238266578627449 ) ) ;
#13744=VERTEX_POINT ( 'NONE', #4144 ) ;
#13750=VERTEX_POINT ( 'NONE', #2665 ) ;
#13759=CIRCLE ( 'NONE', #16453, 15.00000000000000000 ) ;
#13760=CIRCLE ( 'NONE', #14457, 13.99999999999999822 ) ;
#13764=CARTESIAN_POINT ( 'NONE',  ( -15.26367225750305856, 49.50789260602288522, -12.48397009176186145 ) ) ;
#13766=ORIENTED_EDGE ( 'NONE', *, *, #16868, .F. ) ;
#13768=LINE ( 'NONE', #18747, #20180 ) ;
#13788=CARTESIAN_POINT ( 'NONE',  ( -12.02764249544091868, 18.15304305180008271, 11.85355413814486703 ) ) ;
#13796=CARTESIAN_POINT ( 'NONE',  ( -33.48481952675159334, 76.25000000000001421, -2.578432583507806353 ) ) ;
#13822=ORIENTED_EDGE ( 'NONE', *, *, #9402, .T. ) ;
#13833=CARTESIAN_POINT ( 'NONE',  ( -12.23735126049118627, 11.79085703297993248, 11.92262888347531913 ) ) ;
#13835=CARTESIAN_POINT ( 'NONE',  ( -19.71973103665720117, 79.99808926845247470, -12.23885522625830014 ) ) ;
#13862=CARTESIAN_POINT ( 'NONE',  ( -16.66506943655450357, 10.13295816235035751, 12.48647880216494421 ) ) ;
#13866=CARTESIAN_POINT ( 'NONE',  ( -20.29791675083326652, 66.10905085997984543, -2.555169535221540222 ) ) ;
#13870=CARTESIAN_POINT ( 'NONE',  ( -24.22102634534772392, 45.00409005278715568, -9.441307004238941758 ) ) ;
#13872=VECTOR ( 'NONE', #15201, 1000.000000000000000 ) ;
#13874=CARTESIAN_POINT ( 'NONE',  ( -28.49821372255547658, 48.76782331758764855, -0.5569301972970369663 ) ) ;
#13882=CARTESIAN_POINT ( 'NONE',  ( -29.73649742176619881, 50.04042210092456600, -11.28552931171784302 ) ) ;
#13893=EDGE_CURVE ( 'NONE', #3402, #8955, #819, .T. ) ;
#13894=CARTESIAN_POINT ( 'NONE',  ( -15.99999999999999289, 64.25000000000000000, 12.50000000000000000 ) ) ;
#13895=CARTESIAN_POINT ( 'NONE',  ( -28.48915680482256008, 80.00000000000000000, 0.5205403966592370146 ) ) ;
#13897=CARTESIAN_POINT ( 'NONE',  ( -28.48915680482256363, 80.00000000000001421, 0.5205403966592334619 ) ) ;
#13902=CARTESIAN_POINT ( 'NONE',  ( -2.653101600560879625, 65.75000000000000000, 3.131020379152388067 ) ) ;
#13910=EDGE_CURVE ( 'NONE', #16503, #1328, #12750, .T. ) ;
#13913=CIRCLE ( 'NONE', #5099, 4.999999999999995559 ) ;
#13915=ORIENTED_EDGE ( 'NONE', *, *, #12483, .T. ) ;
#13920=AXIS2_PLACEMENT_3D ( 'NONE', #2013, #6549, #8461 ) ;
#13944=CARTESIAN_POINT ( 'NONE',  ( -22.46405759164546367, 79.97811033489706745, -11.66317476315385626 ) ) ;
#13952=AXIS2_PLACEMENT_3D ( 'NONE', #889, #8832, #3637 ) ;
#13955=LINE ( 'NONE', #1613, #15943 ) ;
#13957=EDGE_CURVE ( 'NONE', #11977, #13235, #1432, .T. ) ;
#13977=CARTESIAN_POINT ( 'NONE',  ( -20.99999999999998224, 15.09941697557068530, 11.45643923738960446 ) ) ;
#13982=CIRCLE ( 'NONE', #18036, 17.50000000000000000 ) ;
#13984=CARTESIAN_POINT ( 'NONE',  ( -20.71357962313245693, 45.34957306837157631, -11.59763734586043427 ) ) ;
#13987=CARTESIAN_POINT ( 'NONE',  ( -27.58972166001723636, 58.88968531714240129, 4.685586124710503952 ) ) ;
#13993=ORIENTED_EDGE ( 'NONE', *, *, #17828, .T. ) ;
#13994=ORIENTED_EDGE ( 'NONE', *, *, #17179, .F. ) ;
#13995=CARTESIAN_POINT ( 'NONE',  ( 28.00000000000001066, 65.75000000000001421, -1.525597966175989972 ) ) ;
#13997=CARTESIAN_POINT ( 'NONE',  ( -32.49130957492637606, 50.81462085746833424, -7.575237087458418728 ) ) ;
#14005=CARTESIAN_POINT ( 'NONE',  ( -35.00000000000000000, 65.00000000000000000, -26.49999999999998934 ) ) ;
#14007=CARTESIAN_POINT ( 'NONE',  ( -12.69436033797397201, 18.86475830428287992, 12.05735700452609471 ) ) ;
#14009=LINE ( 'NONE', #12829, #18011 ) ;
#14011=DIRECTION ( 'NONE',  ( 0.000000000000000000, 0.000000000000000000, -1.000000000000000000 ) ) ;
#14019=VERTEX_POINT ( 'NONE', #3488 ) ;
#14021=CARTESIAN_POINT ( 'NONE',  ( -3.195128392259165118, 69.93605911897348903, 1.714708221107726471 ) ) ;
#14042=CARTESIAN_POINT ( 'NONE',  ( -3.905172448840461108, 75.66345017797092964, 3.167069675338881396 ) ) ;
#14045=EDGE_CURVE ( 'NONE', #3287, #19907, #10031, .T. ) ;
#14061=DIRECTION ( 'NONE',  ( 0.000000000000000000, 0.000000000000000000, -1.000000000000000000 ) ) ;
#14067=ORIENTED_EDGE ( 'NONE', *, *, #2660, .F. ) ;
#14072=ORIENTED_EDGE ( 'NONE', *, *, #18084, .F. ) ;
#14084=DIRECTION ( 'NONE',  ( 0.000000000000000000, 0.000000000000000000, -1.000000000000000000 ) ) ;
#14087=CARTESIAN_POINT ( 'NONE',  ( -28.21861819285526352, 49.99051376660081303, -12.54928731108197404 ) ) ;
#14092=CARTESIAN_POINT ( 'NONE',  ( -27.87663165302654633, 46.26680992104923718, -3.912879880524708920 ) ) ;
#14098=CARTESIAN_POINT ( 'NONE',  ( 1.501123442541940634, 76.50873768552941101, -2.871813542384042961 ) ) ;
#14099=ORIENTED_EDGE ( 'NONE', *, *, #15224, .F. ) ;
#14101=CYLINDRICAL_SURFACE ( 'NONE', #10530, 13.99999999999999822 ) ;
#14103=CARTESIAN_POINT ( 'NONE',  ( -33.51303128878281257, 52.95196417805331635, -3.530639089860408308 ) ) ;
#14105=CARTESIAN_POINT ( 'NONE',  ( -28.06703991579542645, 9.091582454895631216, 3.326663291586896776 ) ) ;
#14125=CARTESIAN_POINT ( 'NONE',  ( -15.99999999999999289, 80.00000000000000000, 0.000000000000000000 ) ) ;
#14133=CARTESIAN_POINT ( 'NONE',  ( -3.510843195177425713, 80.00000000000000000, 0.5205403966592461185 ) ) ;
#14149=CARTESIAN_POINT ( 'NONE',  ( 26.99999999999999645, 65.00000000000000000, -12.50000000000000000 ) ) ;
#14151=CARTESIAN_POINT ( 'NONE',  ( -14.99999999999999645, 0.000000000000000000, -15.00000000000000000 ) ) ;
#14152=CARTESIAN_POINT ( 'NONE',  ( -4.674616544174982735, 67.03307707865302234, 5.290582662559626392 ) ) ;
#14183=VECTOR ( 'NONE', #10718, 1000.000000000000000 ) ;
#14184=CARTESIAN_POINT ( 'NONE',  ( -18.51922807846269592, 10.76830012676478709, 12.24661932923539354 ) ) ;
#14187=CARTESIAN_POINT ( 'NONE',  ( -15.99999999999999289, 80.00000000000000000, 0.000000000000000000 ) ) ;
#14198=CARTESIAN_POINT ( 'NONE',  ( -7.283141699791834789, 49.98730520602950378, -8.963927540845297415 ) ) ;
#14207=CARTESIAN_POINT ( 'NONE',  ( -3.599723856067730487, 79.99999999992392929, -1.584264587336005503 ) ) ;
#14210=EDGE_CURVE ( 'NONE', #8547, #11638, #13768, .T. ) ;
#14214=CARTESIAN_POINT ( 'NONE',  ( 1.503428104146816491, 53.42452153058392383, -2.951951819453562997 ) ) ;
#14215=CARTESIAN_POINT ( 'NONE',  ( -34.33329038210762718, 65.74999999999997158, -2.193932927905878127 ) ) ;
#14232=CIRCLE ( 'NONE', #10806, 17.50000000000000000 ) ;
#14239=CARTESIAN_POINT ( 'NONE',  ( -3.082880228654353072, 72.10661837392622431, 0.7232648427671327651 ) ) ;
#14243=EDGE_CURVE ( 'NONE', #9665, #5157, #20629, .T. ) ;
#14258=DIRECTION ( 'NONE',  ( 0.000000000000000000, 0.000000000000000000, -1.000000000000000000 ) ) ;
#14261=CARTESIAN_POINT ( 'NONE',  ( -3.836925286482116171, 76.23982303504118363, 2.898234736985788818 ) ) ;
#14264=CARTESIAN_POINT ( 'NONE',  ( -33.48481952675158624, 76.25000000000001421, -2.578432583507807685 ) ) ;
#14277=AXIS2_PLACEMENT_3D ( 'NONE', #714, #19888, #16926 ) ;
#14282=DIRECTION ( 'NONE',  ( 0.000000000000000000, 0.000000000000000000, -1.000000000000000000 ) ) ;
#14284=CONICAL_SURFACE ( 'NONE', #20684, 14.99999999999999645, 0.7853981633974543852 ) ;
#14293=CARTESIAN_POINT ( 'NONE',  ( 30.10683012259193703, -10.00000000000000000, 0.000000000000000000 ) ) ;
#14300=ORIENTED_EDGE ( 'NONE', *, *, #11000, .T. ) ;
#14303=CARTESIAN_POINT ( 'NONE',  ( -4.526739825310654552, 50.00778237576246710, -13.04232340071289897 ) ) ;
#14317=LINE ( 'NONE', #11113, #20666 ) ;
#14318=CARTESIAN_POINT ( 'NONE',  ( -0.09406327930139435356, 50.50908616029219900, -8.609884709595448271 ) ) ;
#14324=CARTESIAN_POINT ( 'NONE',  ( -0.1607576869230442629, 66.25779166050591584, 2.455816886943473332 ) ) ;
#14333=DIRECTION ( 'NONE',  ( -0.000000000000000000, 1.000000000000000000, -0.000000000000000000 ) ) ;
#14339=EDGE_CURVE ( 'NONE', #3730, #14650, #19265, .T. ) ;
#14343=CARTESIAN_POINT ( 'NONE',  ( -0.003873131613744759151, 68.02992772322234316, 2.199708061508872881 ) ) ;
#14355=CARTESIAN_POINT ( 'NONE',  ( -15.99999999999999289, -9.999999999999994671, -4.999999999999989342 ) ) ;
#14365=DIRECTION ( 'NONE',  ( -0.000000000000000000, -1.000000000000000000, -0.000000000000000000 ) ) ;
#14368=LINE ( 'NONE', #15839, #14911 ) ;
#14370=CARTESIAN_POINT ( 'NONE',  ( -29.33334206987314019, 76.88745196853791697, -3.296735915519156013 ) ) ;
#14371=VECTOR ( 'NONE', #13112, 1000.000000000000000 ) ;
#14372=ORIENTED_EDGE ( 'NONE', *, *, #12651, .T. ) ;
#14373=ORIENTED_EDGE ( 'NONE', *, *, #19788, .F. ) ;
#14377=EDGE_LOOP ( 'NONE', ( #1699, #12524, #16365, #19484, #18146, #2708, #10979, #10768, #9531 ) ) ;
#14379=CARTESIAN_POINT ( 'NONE',  ( -27.46983130148931807, 79.99999999986543742, -4.984538917065587604 ) ) ;
#14384=DIRECTION ( 'NONE',  ( 0.000000000000000000, 0.000000000000000000, 1.000000000000000000 ) ) ;
#14388=DIRECTION ( 'NONE',  ( -0.000000000000000000, -1.000000000000000000, -0.000000000000000000 ) ) ;
#14397=CARTESIAN_POINT ( 'NONE',  ( -46.99999999999998579, 65.00000000000000000, -22.50000000000000000 ) ) ;
#14402=CARTESIAN_POINT ( 'NONE',  ( 1.015643852013114135, 51.37805928129599664, -6.209778783225347709 ) ) ;
#14405=CARTESIAN_POINT ( 'NONE',  ( 30.00000000000000000, 0.000000000000000000, 28.99999999999999645 ) ) ;
#14407=VECTOR ( 'NONE', #2786, 1000.000000000000000 ) ;
#14412=CARTESIAN_POINT ( 'NONE',  ( -5.893702928470589519, 79.63451458383713089, -9.058872303765229006 ) ) ;
#14418=CARTESIAN_POINT ( 'NONE',  ( -31.85787517160000704, 63.46251313055055476, 2.426180918394787334 ) ) ;
#14419=CARTESIAN_POINT ( 'NONE',  ( -28.49950992282111173, 8.571386728324103643, -0.3595220123468740869 ) ) ;
#14421=ORIENTED_EDGE ( 'NONE', *, *, #11869, .T. ) ;
#14431=EDGE_CURVE ( 'NONE', #1521, #15381, #3770, .T. ) ;
#14443=CARTESIAN_POINT ( 'NONE',  ( -0.6518079380778646348, 64.24999999999998579, 2.481238266578627449 ) ) ;
#14457=AXIS2_PLACEMENT_3D ( 'NONE', #10558, #12060, #19786 ) ;
#14472=ORIENTED_EDGE ( 'NONE', *, *, #6963, .F. ) ;
#14479=CARTESIAN_POINT ( 'NONE',  ( -28.59745709644790779, 78.78634076744671688, -6.409256716263459275 ) ) ;
#14489=DIRECTION ( 'NONE',  ( 0.000000000000000000, 0.000000000000000000, -1.000000000000000000 ) ) ;
#14500=CARTESIAN_POINT ( 'NONE',  ( -29.99999999999993605, 5.000000000000018652, -8.526030067124198197 ) ) ;
#14503=ADVANCED_FACE ( 'NONE', ( #5875 ), #19455, .T. ) ;
#14505=CIRCLE ( 'NONE', #5655, 4.999999999999997335 ) ;
#14509=CARTESIAN_POINT ( 'NONE',  ( -11.62985761713838606, 45.38383096773601011, -11.71622545425357842 ) ) ;
#14513=CARTESIAN_POINT ( 'NONE',  ( -25.51376811551812551, 45.02819711329399865, -8.117256888969443196 ) ) ;
#14514=AXIS2_PLACEMENT_3D ( 'NONE', #17196, #20260, #2784 ) ;
#14517=ORIENTED_EDGE ( 'NONE', *, *, #19357, .F. ) ;
#14521=AXIS2_PLACEMENT_3D ( 'NONE', #14149, #7755, #14258 ) ;
#14522=CARTESIAN_POINT ( 'NONE',  ( -5.030706511663012748, 80.00000000026815883, -6.044438231909158077 ) ) ;
#14530=ORIENTED_EDGE ( 'NONE', *, *, #18968, .T. ) ;
#14536=CARTESIAN_POINT ( 'NONE',  ( 30.10683012259193703, 0.000000000000000000, 5.999999999999998224 ) ) ;
#14537=CARTESIAN_POINT ( 'NONE',  ( -27.65382774999337911, 58.21050512791210707, 4.526042831532911315 ) ) ;
#14542=CARTESIAN_POINT ( 'NONE',  ( -29.99999999999999645, -10.00000000000000000, 15.00000000000000000 ) ) ;
#14551=ORIENTED_EDGE ( 'NONE', *, *, #11825, .F. ) ;
#14574=ORIENTED_EDGE ( 'NONE', *, *, #11072, .F. ) ;
#14578=CIRCLE ( 'NONE', #16581, 15.00000000000000000 ) ;
#14579=CARTESIAN_POINT ( 'NONE',  ( -32.02492996559928429, 68.25592811474751898, 2.150873336511315070 ) ) ;
#14583=CARTESIAN_POINT ( 'NONE',  ( -27.40890815691616567, 79.34446119967614663, -7.911977669603216690 ) ) ;
#14588=CARTESIAN_POINT ( 'NONE',  ( -29.99999999999999645, 5.000000000000000000, -30.00000000000000000 ) ) ;
#14594=ORIENTED_EDGE ( 'NONE', *, *, #14431, .F. ) ;
#14600=CARTESIAN_POINT ( 'NONE',  ( -15.99999999999999289, 80.00000000000000000, 0.000000000000000000 ) ) ;
#14605=CARTESIAN_POINT ( 'NONE',  ( -28.35376157792325102, 6.482833755044617341, -1.962836280258419164 ) ) ;
#14608=ORIENTED_EDGE ( 'NONE', *, *, #16615, .T. ) ;
#14616=CARTESIAN_POINT ( 'NONE',  ( -11.02792089128730701, 49.53819989913056077, -11.47781853721724232 ) ) ;
#14619=CARTESIAN_POINT ( 'NONE',  ( -15.99999999999999289, 15.09941697557068530, 0.9999999999999991118 ) ) ;
#14628=CARTESIAN_POINT ( 'NONE',  ( -6.205439792651712416, 80.00000000016144952, -7.778117258980097759 ) ) ;
#14631=ORIENTED_EDGE ( 'NONE', *, *, #20243, .T. ) ;
#14644=AXIS2_PLACEMENT_3D ( 'NONE', #11523, #19375, #1675 ) ;
#14645=AXIS2_PLACEMENT_3D ( 'NONE', #1481, #6026, #4455 ) ;
#14650=VERTEX_POINT ( 'NONE', #13391 ) ;
#14654=EDGE_LOOP ( 'NONE', ( #14834, #20705, #2077, #9703 ) ) ;
#14656=VECTOR ( 'NONE', #12764, 1000.000000000000000 ) ;
#14658=CARTESIAN_POINT ( 'NONE',  ( -0.1730685457077962841, 65.99841087575602216, 2.475388239833483439 ) ) ;
#14666=FACE_BOUND ( 'NONE', #16842, .T. ) ;
#14673=DIRECTION ( 'NONE',  ( 0.000000000000000000, 0.000000000000000000, -1.000000000000000000 ) ) ;
#14679=DIRECTION ( 'NONE',  ( 0.000000000000000000, -0.000000000000000000, 1.000000000000000000 ) ) ;
#14687=CARTESIAN_POINT ( 'NONE',  ( -33.31772531566733164, 74.84505238333375132, -1.139833306050677564 ) ) ;
#14690=CARTESIAN_POINT ( 'NONE',  ( -29.47382129635126802, 77.46132694877815084, -4.041171758127458880 ) ) ;
#14696=CARTESIAN_POINT ( 'NONE',  ( -28.75894515448919364, 64.25000000000001421, 3.522626389267836000 ) ) ;
#14697=VERTEX_POINT ( 'NONE', #13290 ) ;
#14705=ORIENTED_EDGE ( 'NONE', *, *, #20551, .T. ) ;
#14710=CARTESIAN_POINT ( 'NONE',  ( -26.39516425332331195, 9.975807959609232611, -6.950086042755424742 ) ) ;
#14719=CARTESIAN_POINT ( 'NONE',  ( -3.180065357767781098, 59.84479038527697980, 1.598284787553928776 ) ) ;
#14720=CARTESIAN_POINT ( 'NONE',  ( -14.13423450066001585, 79.99988027213446173, -12.43461861220364817 ) ) ;
#14723=B_SPLINE_CURVE_WITH_KNOTS ( 'NONE', 3,
 ( #13579, #1810, #14765, #6764, #11560, #14868, #9942, #16541, #19707, #18129, #13155, #10047, #18028, #13261 ),
 .UNSPECIFIED., .F., .F.,
 ( 4, 2, 2, 2, 2, 2, 4 ),
 ( 0.000000000000000000, 0.001404861450950249668, 0.002107292176425374503, 0.002809722901900499337, 0.003512153627375624605, 0.004214584352850749005, 0.005619445803801009082 ),
 .UNSPECIFIED. ) ;
#14731=EDGE_CURVE ( 'NONE', #4880, #3383, #3837, .T. ) ;
#14745=ADVANCED_FACE ( 'NONE', ( #662 ), #7119, .F. ) ;
#14747=CARTESIAN_POINT ( 'NONE',  ( -27.30676186341464273, 66.39265442260771977, 5.329868606387897501 ) ) ;
#14753=EDGE_CURVE ( 'NONE', #1893, #6192, #15769, .T. ) ;
#14759=EDGE_CURVE ( 'NONE', #5157, #7840, #12222, .T. ) ;
#14763=ORIENTED_EDGE ( 'NONE', *, *, #4437, .T. ) ;
#14765=CARTESIAN_POINT ( 'NONE',  ( -27.76006405428915613, 65.74999999999997158, 4.526879896143035431 ) ) ;
#14769=ADVANCED_FACE ( 'NONE', ( #18790, #2682, #5840, #9227 ), #4162, .T. ) ;
#14772=AXIS2_PLACEMENT_3D ( 'NONE', #3784, #16728, #15160 ) ;
#14773=VERTEX_POINT ( 'NONE', #776 ) ;
#14780=CARTESIAN_POINT ( 'NONE',  ( 30.00000000000000000, -10.00000000000000000, 28.99999999999999645 ) ) ;
#14792=CARTESIAN_POINT ( 'NONE',  ( -31.21251268849638194, 78.92002130297235851, -6.902655774462157723 ) ) ;
#14806=ADVANCED_FACE ( 'NONE', ( #1193 ), #20577, .F. ) ;
#14807=ORIENTED_EDGE ( 'NONE', *, *, #10976, .T. ) ;
#14812=( BOUNDED_SURFACE ( )  B_SPLINE_SURFACE ( 3, 2, ( 
 ( #7998, #6504, #8093 ),
 ( #16386, #11299, #19762 ),
 ( #14710, #8413, #19443 ),
 ( #14913, #1861, #8307 ),
 ( #17769, #6400, #14500 ),
 ( #3141, #20927, #9587 ),
 ( #19653, #6709, #3236 ),
 ( #16085, #5129, #11614 ),
 ( #18078, #69, #1553 ),
 ( #9691, #16482, #12898 ),
 ( #1964, #1653, #13314 ),
 ( #4925, #14605, #11194 ),
 ( #11400, #15342, #17015 ),
 ( #2496, #4072, #7248 ),
 ( #15234, #16587, #3969 ),
 ( #19861, #796, #10097 ),
 ( #18499, #11717, #10419 ),
 ( #15441, #2383, #20185 ),
 ( #18280, #13732, #5227 ),
 ( #900, #12036, #5647 ),
 ( #7141, #5328, #18180 ),
 ( #12137, #8529, #3752 ),
 ( #2280, #11819, #15028 ),
 ( #20083, #487, #6927 ),
 ( #10208, #2180, #16701 ),
 ( #8632, #15130, #585 ),
 ( #11933, #19966, #5432 ),
 ( #18393, #3862, #10311 ) ),
 .UNSPECIFIED., .F., .F., .F. ) 
 B_SPLINE_SURFACE_WITH_KNOTS ( ( 4, 2, 2, 2, 2, 2, 2, 2, 2, 2, 2, 2, 2, 4 ),
 ( 3, 3 ),
 ( 0.009371192738994881324, 0.01079808352755677603, 0.01222497431611867247, 0.01365186510468056891, 0.01507875589324246535, 0.01793253747036625823, 0.01935942825892815466, 0.02078631904749004763, 0.02221320983605194060, 0.02364010062461383704, 0.02649388220173762992, 0.02934766377886142280, 0.03077455456742331924, 0.03220144535598521568 ),
 ( 0.000000000000000000, 1.000000000000000000 ),
 .UNSPECIFIED. ) 
 GEOMETRIC_REPRESENTATION_ITEM ( )  RATIONAL_B_SPLINE_SURFACE ( (
 ( 1.000000000000000000, 0.7071067811865479058, 1.000000000000000000),
 ( 1.000000000000000000, 0.7232527279161264921, 1.000000000000000000),
 ( 1.000000000000000000, 0.7388286583289560561, 1.000000000000000000),
 ( 1.000000000000000000, 0.7685446699867291009, 1.000000000000000000),
 ( 1.000000000000000000, 0.7826850257046925607, 1.000000000000000000),
 ( 1.000000000000000000, 0.8093023715178216948, 1.000000000000000000),
 ( 1.000000000000000000, 0.8217945561033374036, 1.000000000000000000),
 ( 1.000000000000000000, 0.8445755018420567639, 1.000000000000000000),
 ( 1.000000000000000000, 0.8549247766998627762, 1.000000000000000000),
 ( 1.000000000000000000, 0.8828010807230063373, 1.000000000000000000),
 ( 1.000000000000000000, 0.8971838639936082771, 1.000000000000000000),
 ( 1.000000000000000000, 0.9119221572953989385, 1.000000000000000000),
 ( 1.000000000000000000, 0.9157004699627206978, 1.000000000000000000),
 ( 1.000000000000000000, 0.9207044786150797577, 1.000000000000000000),
 ( 1.000000000000000000, 0.9219484747058886986, 1.000000000000000000),
 ( 1.000000000000000000, 0.9219603739042575574, 1.000000000000000000),
 ( 1.000000000000000000, 0.9207283435489677093, 1.000000000000000000),
 ( 1.000000000000000000, 0.9158001944594933441, 1.000000000000000000),
 ( 1.000000000000000000, 0.9120921721005434968, 1.000000000000000000),
 ( 1.000000000000000000, 0.8973220332527075405, 1.000000000000000000),
 ( 1.000000000000000000, 0.8828883913922480620, 1.000000000000000000),
 ( 1.000000000000000000, 0.8457423740019180958, 1.000000000000000000),
 ( 1.000000000000000000, 0.8230077850553781937, 1.000000000000000000),
 ( 1.000000000000000000, 0.7829299428437686004, 1.000000000000000000),
 ( 1.000000000000000000, 0.7686927448236463567, 1.000000000000000000),
 ( 1.000000000000000000, 0.7388689099750124223, 1.000000000000000000),
 ( 1.000000000000000000, 0.7232573842950190679, 1.000000000000000000),
 ( 1.000000000000000000, 0.7071067811865474617, 1.000000000000000000) ) ) 
 REPRESENTATION_ITEM ( '' )  SURFACE ( )  );
#14813=DIRECTION ( 'NONE',  ( -0.000000000000000000, -1.000000000000000000, -0.000000000000000000 ) ) ;
#14816=ORIENTED_EDGE ( 'NONE', *, *, #8777, .F. ) ;
#14821=ORIENTED_EDGE ( 'NONE', *, *, #5970, .T. ) ;
#14823=CARTESIAN_POINT ( 'NONE',  ( -3.812720765152911806, 52.63858550657156599, -3.991166449876146327 ) ) ;
#14824=CARTESIAN_POINT ( 'NONE',  ( -12.28221561448063781, 79.99809398375025182, -12.23915253492440947 ) ) ;
#14829=VERTEX_POINT ( 'NONE', #17304 ) ;
#14834=ORIENTED_EDGE ( 'NONE', *, *, #14753, .T. ) ;
#14851=CARTESIAN_POINT ( 'NONE',  ( -27.62855338901809787, 51.88754995109739099, -5.120729935976574332 ) ) ;
#14852=CARTESIAN_POINT ( 'NONE',  ( -19.30416908549006649, 18.86621361051762591, 12.05778820527624262 ) ) ;
#14853=AXIS2_PLACEMENT_3D ( 'NONE', #1102, #17417, #17628 ) ;
#14863=CIRCLE ( 'NONE', #9064, 5.999999999999998224 ) ;
#14868=CARTESIAN_POINT ( 'NONE',  ( -28.75604140624042770, 65.74999999999997158, 3.524958307384044698 ) ) ;
#14874=EDGE_CURVE ( 'NONE', #1492, #15273, #20783, .T. ) ;
#14875=ORIENTED_EDGE ( 'NONE', *, *, #12429, .F. ) ;
#14895=CARTESIAN_POINT ( 'NONE',  ( -26.76057640522419590, 79.79422864173648122, -10.01493943371489159 ) ) ;
#14898=ORIENTED_EDGE ( 'NONE', *, *, #15660, .F. ) ;
#14907=ORIENTED_EDGE ( 'NONE', *, *, #17876, .F. ) ;
#14908=LINE ( 'NONE', #8836, #11558 ) ;
#14910=CARTESIAN_POINT ( 'NONE',  ( -32.77319314005540463, 77.96684442108207236, -4.956410556015048208 ) ) ;
#14911=VECTOR ( 'NONE', #12863, 1000.000000000000000 ) ;
#14913=CARTESIAN_POINT ( 'NONE',  ( -26.75388419629425130, 9.893953324963231211, -6.380996046697354096 ) ) ;
#14922=CARTESIAN_POINT ( 'NONE',  ( -3.058993387607990666, 55.97632480169432512, -0.5003277293098231659 ) ) ;
#14923=CARTESIAN_POINT ( 'NONE',  ( -1.033406382133238655, 79.01409684087832375, -7.140683506250414148 ) ) ;
#14931=CARTESIAN_POINT ( 'NONE',  ( -15.99999999999999289, 10.09941697557069418, 4.999999999999989342 ) ) ;
#14952=CARTESIAN_POINT ( 'NONE',  ( -33.46931044135702393, 53.99090883974105282, -2.305310864414939598 ) ) ;
#14958=ORIENTED_EDGE ( 'NONE', *, *, #3416, .F. ) ;
#14989=VECTOR ( 'NONE', #10081, 1000.000000000000000 ) ;
#14994=CARTESIAN_POINT ( 'NONE',  ( -12.79128543553366093, 69.99684855425128660, -3.836613224171032233 ) ) ;
#15004=CARTESIAN_POINT ( 'NONE',  ( -19.59011831531341841, 79.99589872796802581, -12.11680902303608853 ) ) ;
#15012=LINE ( 'NONE', #10084, #19868 ) ;
#15014=ORIENTED_EDGE ( 'NONE', *, *, #324, .T. ) ;
#15018=CARTESIAN_POINT ( 'NONE',  ( -9.243941288027137659, 79.99999999991588595, -10.56315151873520541 ) ) ;
#15025=ADVANCED_FACE ( 'NONE', ( #13474 ), #223, .F. ) ;
#15028=CARTESIAN_POINT ( 'NONE',  ( -30.00000000000011369, 4.999999999999960920, 7.262422089269331416 ) ) ;
#15031=ORIENTED_EDGE ( 'NONE', *, *, #17548, .T. ) ;
#15034=CARTESIAN_POINT ( 'NONE',  ( -5.147701114615496287, 45.33223473607662157, -6.247204070674920118 ) ) ;
#15038=CARTESIAN_POINT ( 'NONE',  ( -3.126021133370410432, 54.92993604554487064, -1.368878731129744564 ) ) ;
#15039=CARTESIAN_POINT ( 'NONE',  ( -2.078177106580701317, 79.32247413568823902, -8.032153923986145472 ) ) ;
#15059=DIRECTION ( 'NONE',  ( 0.000000000000000000, 0.000000000000000000, 1.000000000000000000 ) ) ;
#15062=CARTESIAN_POINT ( 'NONE',  ( -28.49184912364534839, 49.99505663536145050, 0.5228165434693862190 ) ) ;
#15066=( BOUNDED_CURVE ( )  B_SPLINE_CURVE ( 3, ( #19780, #13020, #2093, #14931 ),
 .UNSPECIFIED., .F., .F. ) 
 B_SPLINE_CURVE_WITH_KNOTS ( ( 4, 4 ),
 ( 1.772154247585230769, 3.141592653589793116 ),
 .UNSPECIFIED. ) 
 CURVE ( )  GEOMETRIC_REPRESENTATION_ITEM ( )  RATIONAL_B_SPLINE_CURVE ( ( 1.000000000000000000, 0.8497311128276563430, 0.8497311128276563430, 1.000000000000000000 ) ) 
 REPRESENTATION_ITEM ( '' )  );
#15074=LINE ( 'NONE', #15283, #1388 ) ;
#15087=LINE ( 'NONE', #6990, #18813 ) ;
#15090=FACE_OUTER_BOUND ( 'NONE', #5776, .T. ) ;
#15104=CARTESIAN_POINT ( 'NONE',  ( -25.51565122030220323, 79.99999999992057553, -8.118105310439162281 ) ) ;
#15108=EDGE_CURVE ( 'NONE', #8219, #15321, #9971, .T. ) ;
#15113=CARTESIAN_POINT ( 'NONE',  ( -30.88448036966982002, 64.25000000000000000, 2.547625675852274618 ) ) ;
#15114=ORIENTED_EDGE ( 'NONE', *, *, #11072, .T. ) ;
#15120=CARTESIAN_POINT ( 'NONE',  ( -3.212349491796369527, 78.65050410969293182, -6.103909342517296999 ) ) ;
#15126=AXIS2_PLACEMENT_3D ( 'NONE', #1487, #17710, #19290 ) ;
#15127=CARTESIAN_POINT ( 'NONE',  ( -33.43925266485176451, 76.85164673649258305, -3.302532775402095222 ) ) ;
#15130=CARTESIAN_POINT ( 'NONE',  ( -26.22900660273689155, 5.421942632918632654, 7.194350572235736152 ) ) ;
#15140=CARTESIAN_POINT ( 'NONE',  ( -4.675102993692958897, 62.87218805480786443, 5.292445494479565582 ) ) ;
#15142=AXIS2_PLACEMENT_3D ( 'NONE', #10720, #20371, #16882 ) ;
#15147=EDGE_CURVE ( 'NONE', #20014, #15175, #3910, .T. ) ;
#15148=ORIENTED_EDGE ( 'NONE', *, *, #14874, .T. ) ;
#15160=DIRECTION ( 'NONE',  ( 1.000000000000000000, 0.000000000000000000, 0.000000000000000000 ) ) ;
#15167=CARTESIAN_POINT ( 'NONE',  ( -30.91092412438536385, 50.20590819142025651, -10.00467867777946473 ) ) ;
#15168=CARTESIAN_POINT ( 'NONE',  ( -16.66469718191209282, 20.06594084399080558, 12.48650452048989479 ) ) ;
#15173=ADVANCED_BREP_SHAPE_REPRESENTATION ( '', ( #3293, #18233 ), #6025 ) ;
#15174=ORIENTED_EDGE ( 'NONE', *, *, #5494, .T. ) ;
#15175=VERTEX_POINT ( 'NONE', #9016 ) ;
#15180=CARTESIAN_POINT ( 'NONE',  ( -4.701390418375632763, 64.25000000000000000, 5.347094680480811490 ) ) ;
#15195=DIRECTION ( 'NONE',  ( -1.000000000000000000, 0.000000000000000000, -0.000000000000000000 ) ) ;
#15201=DIRECTION ( 'NONE',  ( -0.000000000000000000, -0.000000000000000000, 1.000000000000000000 ) ) ;
#15210=CARTESIAN_POINT ( 'NONE',  ( -18.59213065175719493, 79.99957779460252993, -12.37049764041025135 ) ) ;
#15221=CARTESIAN_POINT ( 'NONE',  ( -3.510843195177425713, 80.00000000000000000, 0.5205403966592460074 ) ) ;
#15224=EDGE_CURVE ( 'NONE', #1288, #13189, #6258, .T. ) ;
#15225=EDGE_LOOP ( 'NONE', ( #2884, #9038, #4966 ) ) ;
#15234=CARTESIAN_POINT ( 'NONE',  ( -28.49993446417160570, 8.570804147430656883, -0.3390835457399271058 ) ) ;
#15241=ORIENTED_EDGE ( 'NONE', *, *, #8626, .F. ) ;
#15244=DIRECTION ( 'NONE',  ( -0.000000000000000000, 1.000000000000000000, -0.000000000000000000 ) ) ;
#15250=ORIENTED_EDGE ( 'NONE', *, *, #422, .F. ) ;
#15251=ORIENTED_EDGE ( 'NONE', *, *, #15754, .F. ) ;
#15257=DIRECTION ( 'NONE',  ( 0.000000000000000000, -1.000000000000000000, 0.000000000000000000 ) ) ;
#15260=ORIENTED_EDGE ( 'NONE', *, *, #583, .F. ) ;
#15270=CARTESIAN_POINT ( 'NONE',  ( -27.10521411282678628, 51.35483501200679513, -5.980665530051757273 ) ) ;
#15273=VERTEX_POINT ( 'NONE', #7639 ) ;
#15283=CARTESIAN_POINT ( 'NONE',  ( -14.99999999999999645, 5.000000000000000000, 30.00000000000000000 ) ) ;
#15294=DIRECTION ( 'NONE',  ( 0.000000000000000000, 0.000000000000000000, -1.000000000000000000 ) ) ;
#15297=DIRECTION ( 'NONE',  ( 1.000000000000000000, 0.000000000000000000, 0.000000000000000000 ) ) ;
#15302=CARTESIAN_POINT ( 'NONE',  ( -28.18912803645524789, 76.46633113979225982, 2.786148689273399981 ) ) ;
#15303=DIRECTION ( 'NONE',  ( 0.000000000000000000, 0.000000000000000000, -1.000000000000000000 ) ) ;
#15318=CARTESIAN_POINT ( 'NONE',  ( -16.52214040532013684, 80.00000000000014211, -12.49180211257053230 ) ) ;
#15321=VERTEX_POINT ( 'NONE', #11251 ) ;
#15329=LINE ( 'NONE', #12232, #18630 ) ;
#15333=ORIENTED_EDGE ( 'NONE', *, *, #13010, .T. ) ;
#15335=EDGE_LOOP ( 'NONE', ( #16186, #11321, #4790, #18215 ) ) ;
#15342=CARTESIAN_POINT ( 'NONE',  ( -28.40887611229263143, 6.478901333902477688, -1.571843926571936612 ) ) ;
#15373=EDGE_CURVE ( 'NONE', #15175, #4315, #20670, .T. ) ;
#15375=CARTESIAN_POINT ( 'NONE',  ( -18.57755300701755274, 49.50817056232955338, -12.23824556917615780 ) ) ;
#15377=EDGE_CURVE ( 'NONE', #14697, #15381, #17463, .T. ) ;
#15381=VERTEX_POINT ( 'NONE', #17507 ) ;
#15398=PLANE ( 'NONE',  #10104 ) ;
#15402=DIRECTION ( 'NONE',  ( 0.000000000000000000, -1.000000000000000000, 0.000000000000000000 ) ) ;
#15404=CARTESIAN_POINT ( 'NONE',  ( -27.70576433140186268, 72.30161019874638839, 4.406123080992779606 ) ) ;
#15428=CARTESIAN_POINT ( 'NONE',  ( -4.318268741000043320, 72.07281518094384865, 4.467622400254039228 ) ) ;
#15429=B_SPLINE_CURVE_WITH_KNOTS ( 'NONE', 3,
 ( #2163, #8616, #15113, #569, #12988, #16262, #1743, #13194, #14696, #151, #20269, #10510, #18481, #10401 ),
 .UNSPECIFIED., .F., .F.,
 ( 4, 2, 2, 2, 2, 2, 4 ),
 ( 0.000000000000000000, 0.001404842194932282235, 0.002107263292398423027, 0.002809684389864564470, 0.003512105487330705912, 0.004214526584796846054, 0.005619368779729120265 ),
 .UNSPECIFIED. ) ;
#15435=EDGE_LOOP ( 'NONE', ( #14072, #5104 ) ) ;
#15441=CARTESIAN_POINT ( 'NONE',  ( -28.43238653473407496, 8.661473207178586264, 1.341288757007061516 ) ) ;
#15460=VECTOR ( 'NONE', #19110, 1000.000000000000000 ) ;
#15467=DIRECTION ( 'NONE',  ( 0.000000000000000000, 0.000000000000000000, -1.000000000000000000 ) ) ;
#15471=CONICAL_SURFACE ( 'NONE', #894, 14.00000000000000178, 0.7853981633974509435 ) ;
#15475=CARTESIAN_POINT ( 'NONE',  ( -15.63876350448106223, 49.50806937060298196, -12.50030949268231062 ) ) ;
#15481=ORIENTED_EDGE ( 'NONE', *, *, #1391, .F. ) ;
#15483=CARTESIAN_POINT ( 'NONE',  ( 30.00000000000000355, 0.000000000000000000, -28.99999999999999645 ) ) ;
#15484=CARTESIAN_POINT ( 'NONE',  ( -33.99999999999997868, 65.00000000000000000, -12.50000000000000000 ) ) ;
#15485=ORIENTED_EDGE ( 'NONE', *, *, #15924, .T. ) ;
#15489=CARTESIAN_POINT ( 'NONE',  ( 0.7736121223987986184, 51.05006296119952225, -6.934240817527092204 ) ) ;
#15496=( BOUNDED_SURFACE ( )  B_SPLINE_SURFACE ( 3, 2, ( 
 ( #14264, #10956, #16155 ),
 ( #6172, #8063, #18911 ),
 ( #4384, #17320, #12662 ),
 ( #2803, #11060, #1420 ),
 ( #7869, #14370, #12875 ),
 ( #17856, #3119, #44 ),
 ( #20905, #16068, #1630 ),
 ( #9770, #6482, #13185 ),
 ( #8282, #14690, #6379 ),
 ( #19330, #6585, #13085 ),
 ( #20806, #1840, #19234 ),
 ( #19528, #7878, #5002 ),
 ( #14792, #8074, #17538 ),
 ( #9458, #12983, #1429 ),
 ( #4806, #14479, #14379 ),
 ( #17647, #6278, #12771 ),
 ( #4700, #14583, #11169 ),
 ( #17751, #9570, #3216 ),
 ( #14895, #563, #15104 ),
 ( #3836, #10287, #3944 ),
 ( #5524, #10076, #3624 ),
 ( #8817, #18473, #7011 ),
 ( #8392, #11797, #11693 ),
 ( #9966, #18371, #7225 ),
 ( #1944, #355, #11589 ),
 ( #19736, #5412, #18159 ),
 ( #16460, #15004, #16567 ),
 ( #15210, #13498, #19944 ),
 ( #2256, #2360, #11907 ),
 ( #16674, #461, #661 ),
 ( #12011, #6802, #10390 ),
 ( #13288, #16881, #15318 ),
 ( #774, #2049, #3726 ),
 ( #8501, #18058, #6905 ) ),
 .UNSPECIFIED., .F., .F., .T. ) 
 B_SPLINE_SURFACE_WITH_KNOTS ( ( 4, 2, 2, 2, 2, 2, 2, 2, 2, 2, 2, 2, 2, 2, 2, 2, 4 ),
 ( 3, 3 ),
 ( 0.01278509310405299623, 0.01434830319407979539, 0.01591151328410659455, 0.01669311832911999499, 0.01747472337413339197, 0.01903793346416018939, 0.02060114355418698681, 0.02216435364421378423, 0.02529077382426737908, 0.02685398391429417650, 0.02841719400432097392, 0.03154361418437456877, 0.03310682427440136966, 0.03467003436442817055, 0.03623324445445497144, 0.03701484949946837189, 0.03779645454448176539 ),
 ( 0.000000000000000000, 1.000000000000000000 ),
 .UNSPECIFIED. ) 
 GEOMETRIC_REPRESENTATION_ITEM ( )  RATIONAL_B_SPLINE_SURFACE ( (
 ( 1.000000000000000000, 0.7167790485004659207, 1.000000000000000000),
 ( 1.000000000000000000, 0.7293845257053636066, 1.000000000000000000),
 ( 1.000000000000000000, 0.7423068803281102079, 1.000000000000000000),
 ( 1.000000000000000000, 0.7686138469776572224, 1.000000000000000000),
 ( 1.000000000000000000, 0.7816781719490264457, 1.000000000000000000),
 ( 1.000000000000000000, 0.8009424076554686467, 1.000000000000000000),
 ( 1.000000000000000000, 0.8073105603345962500, 1.000000000000000000),
 ( 1.000000000000000000, 0.8199112611634222780, 1.000000000000000000),
 ( 1.000000000000000000, 0.8261570471472956534, 1.000000000000000000),
 ( 1.000000000000000000, 0.8443914605100442117, 1.000000000000000000),
 ( 1.000000000000000000, 0.8559617003901804910, 1.000000000000000000),
 ( 1.000000000000000000, 0.8778584927324852849, 1.000000000000000000),
 ( 1.000000000000000000, 0.8881844774554348287, 1.000000000000000000),
 ( 1.000000000000000000, 0.9075144288648713253, 1.000000000000000000),
 ( 1.000000000000000000, 0.9165151951640571060, 1.000000000000000000),
 ( 1.000000000000000000, 0.9409273377063475108, 1.000000000000000000),
 ( 1.000000000000000000, 0.9539926103734300833, 1.000000000000000000),
 ( 1.000000000000000000, 0.9694264545131714428, 1.000000000000000000),
 ( 1.000000000000000000, 0.9738877056527739384, 1.000000000000000000),
 ( 1.000000000000000000, 0.9815112523102276221, 1.000000000000000000),
 ( 1.000000000000000000, 0.9846522094487469845, 1.000000000000000000),
 ( 1.000000000000000000, 0.9924326897349095011, 1.000000000000000000),
 ( 1.000000000000000000, 0.9954310229819894884, 1.000000000000000000),
 ( 1.000000000000000000, 0.9981072485120531246, 1.000000000000000000),
 ( 1.000000000000000000, 0.9986952519232461523, 1.000000000000000000),
 ( 1.000000000000000000, 0.9994860253291804053, 1.000000000000000000),
 ( 1.000000000000000000, 0.9996937099786900038, 1.000000000000000000),
 ( 1.000000000000000000, 0.9999366964164366767, 1.000000000000000000),
 ( 1.000000000000000000, 0.9999724247964512092, 1.000000000000000000),
 ( 1.000000000000000000, 0.9999959980224297773, 1.000000000000000000),
 ( 1.000000000000000000, 0.9999982534776523657, 1.000000000000000000),
 ( 1.000000000000000000, 1.000000247701407607, 1.000000000000000000),
 ( 1.000000000000000000, 1.000000000000000000, 1.000000000000000000),
 ( 1.000000000000000000, 1.000000000000000000, 1.000000000000000000) ) ) 
 REPRESENTATION_ITEM ( '' )  SURFACE ( )  );
#15505=CARTESIAN_POINT ( 'NONE',  ( -15.99999999999999289, 5.000000000000000000, 0.000000000000000000 ) ) ;
#15525=CARTESIAN_POINT ( 'NONE',  ( 30.00000000000000000, 0.000000000000000000, 15.00000000000000000 ) ) ;
#15537=CARTESIAN_POINT ( 'NONE',  ( -3.544689826710143432, 78.99734867018932505, 1.332611642696186927 ) ) ;
#15544=CARTESIAN_POINT ( 'NONE',  ( -15.34250122215976653, 10.13184782583976684, 12.48692088216763985 ) ) ;
#15555=ORIENTED_EDGE ( 'NONE', *, *, #369, .T. ) ;
#15565=ORIENTED_EDGE ( 'NONE', *, *, #3319, .F. ) ;
#15567=CARTESIAN_POINT ( 'NONE',  ( -20.74074359463745765, 13.47737252516389184, 11.56691115307346251 ) ) ;
#15575=CARTESIAN_POINT ( 'NONE',  ( -23.33357341442864197, 49.70767121013135892, -10.13114767712223951 ) ) ;
#15586=ORIENTED_EDGE ( 'NONE', *, *, #12651, .F. ) ;
#15587=LINE ( 'NONE', #7611, #19674 ) ;
#15589=CARTESIAN_POINT ( 'NONE',  ( -31.27810441140633202, 50.29222651548906953, -9.535589147757439932 ) ) ;
#15590=CARTESIAN_POINT ( 'NONE',  ( 44.00000000000000000, -10.00000000000000000, -15.00000000000000355 ) ) ;
#15600=CYLINDRICAL_SURFACE ( 'NONE', #16015, 5.999999999999998224 ) ;
#15608=ORIENTED_EDGE ( 'NONE', *, *, #11119, .T. ) ;
#15612=ORIENTED_EDGE ( 'NONE', *, *, #15899, .T. ) ;
#15613=VERTEX_POINT ( 'NONE', #12184 ) ;
#15614=CARTESIAN_POINT ( 'NONE',  ( -4.498188040268487953, 64.25000000000001421, 4.917720511238719894 ) ) ;
#15623=VERTEX_POINT ( 'NONE', #15180 ) ;
#15624=LINE ( 'NONE', #20678, #14183 ) ;
#15641=CARTESIAN_POINT ( 'NONE',  ( -14.95727968274949404, 79.99998834348832588, -12.47960036978351894 ) ) ;
#15652=CARTESIAN_POINT ( 'NONE',  ( -34.33334827330879335, 65.74999999999997158, 2.147472525011942857 ) ) ;
#15654=VECTOR ( 'NONE', #16212, 1000.000000000000000 ) ;
#15657=CARTESIAN_POINT ( 'NONE',  ( -34.00000000000000711, 65.00000000000000000, -12.50000000000000000 ) ) ;
#15660=EDGE_CURVE ( 'NONE', #11812, #2307, #949, .T. ) ;
#15663=( GEOMETRIC_REPRESENTATION_CONTEXT ( 3 ) GLOBAL_UNCERTAINTY_ASSIGNED_CONTEXT ( ( #17850 ) ) GLOBAL_UNIT_ASSIGNED_CONTEXT ( ( #19126, #6175, #19324 ) ) REPRESENTATION_CONTEXT ( 'NONE', 'WORKASPACE' ) );
#15666=AXIS2_PLACEMENT_3D ( 'NONE', #17500, #2873, #12322 ) ;
#15674=CARTESIAN_POINT ( 'NONE',  ( -19.05738717796882398, 11.12984937779420136, 12.12347222335699826 ) ) ;
#15677=EDGE_CURVE ( 'NONE', #4564, #4238, #7935, .T. ) ;
#15680=VERTEX_POINT ( 'NONE', #15590 ) ;
#15685=CARTESIAN_POINT ( 'NONE',  ( -25.30425913992641185, 50.18878380057854116, -8.354022865946610921 ) ) ;
#15694=CARTESIAN_POINT ( 'NONE',  ( -2.666657930126863363, 76.88745196853420794, -3.296735915517357451 ) ) ;
#15695=VERTEX_POINT ( 'NONE', #1057 ) ;
#15699=CARTESIAN_POINT ( 'NONE',  ( -28.53155540363584208, 49.99238495923260928, -12.31184910487761996 ) ) ;
#15700=CARTESIAN_POINT ( 'NONE',  ( -28.48501876579843639, 8.591569706101985560, -0.7004361938144425537 ) ) ;
#15703=ORIENTED_EDGE ( 'NONE', *, *, #9772, .T. ) ;
#15704=DIRECTION ( 'NONE',  ( 0.000000000000000000, -1.000000000000000000, 0.000000000000000000 ) ) ;
#15715=CARTESIAN_POINT ( 'NONE',  ( -27.42580490583086572, 69.03990363093173244, 5.071150534606303495 ) ) ;
#15731=ADVANCED_FACE ( 'NONE', ( #7716 ), #15471, .T. ) ;
#15733=DIRECTION ( 'NONE',  ( 0.000000000000000000, -1.000000000000000000, 0.000000000000000000 ) ) ;
#15741=FACE_OUTER_BOUND ( 'NONE', #14654, .T. ) ;
#15744=ORIENTED_EDGE ( 'NONE', *, *, #13957, .T. ) ;
#15752=ORIENTED_EDGE ( 'NONE', *, *, #9229, .F. ) ;
#15754=EDGE_CURVE ( 'NONE', #2330, #4222, #6649, .T. ) ;
#15758=ADVANCED_FACE ( 'NONE', ( #10901 ), #4233, .F. ) ;
#15760=DIRECTION ( 'NONE',  ( 1.000000000000000000, -0.000000000000000000, -0.000000000000000000 ) ) ;
#15769=CIRCLE ( 'NONE', #8631, 13.99999999999999822 ) ;
#15780=EDGE_CURVE ( 'NONE', #3348, #4596, #1128, .T. ) ;
#15782=CARTESIAN_POINT ( 'NONE',  ( -8.667048942563669200, 49.69984668619762402, -10.14481273401418449 ) ) ;
#15797=CARTESIAN_POINT ( 'NONE',  ( -30.29050950868652237, 50.09228121850021154, -10.73328253952971778 ) ) ;
#15806=( LENGTH_UNIT ( ) NAMED_UNIT ( * ) SI_UNIT ( .MILLI., .METRE. ) );
#15837=CIRCLE ( 'NONE', #1605, 12.50000000000000000 ) ;
#15839=CARTESIAN_POINT ( 'NONE',  ( 45.00000000000000000, 5.000000000000000000, 0.000000000000000000 ) ) ;
#15841=CARTESIAN_POINT ( 'NONE',  ( -20.90625477759164141, 14.43164562092441372, 0.9643584936165373600 ) ) ;
#15845=ORIENTED_EDGE ( 'NONE', *, *, #20711, .F. ) ;
#15846=CARTESIAN_POINT ( 'NONE',  ( -11.16244655246401152, 13.79331584593744431, 11.52618815104203165 ) ) ;
#15848=DIRECTION ( 'NONE',  ( 0.000000000000000000, 0.000000000000000000, -1.000000000000000000 ) ) ;
#15868=DIRECTION ( 'NONE',  ( 0.000000000000000000, 0.000000000000000000, -1.000000000000000000 ) ) ;
#15879=CARTESIAN_POINT ( 'NONE',  ( -10.08519122218491404, 49.57845857190523731, -11.02153694242965187 ) ) ;
#15886=B_SPLINE_CURVE_WITH_KNOTS ( 'NONE', 3,
 ( #5296, #19514, #11788, #16557, #3715, #13278, #18251, #10169, #14994, #8488, #16665, #6786, #17844, #5195, #8173, #6574, #2146, #13073, #8597, #1723, #9956, #16448 ),
 .UNSPECIFIED., .F., .F.,
 ( 4, 2, 2, 2, 2, 2, 2, 2, 2, 2, 4 ),
 ( 0.000000000000000000, 0.002138836336596501835, 0.003208254504894771618, 0.004277672673193041834, 0.004812381757342193422, 0.005347090841491346745, 0.006416509009789626503, 0.006951218093938767682, 0.007485927178087907995, 0.008020636262237049174, 0.008555345346386189487 ),
 .UNSPECIFIED. ) ;
#15890=CARTESIAN_POINT ( 'NONE',  ( -3.671937341326915849, 79.99999999995419842, -2.072940693968563064 ) ) ;
#15893=DIRECTION ( 'NONE',  ( -0.000000000000000000, -1.000000000000000000, -0.000000000000000000 ) ) ;
#15895=CARTESIAN_POINT ( 'NONE',  ( 1.475260119819425508, 52.70730118409597509, -3.895249003718037617 ) ) ;
#15896=CARTESIAN_POINT ( 'NONE',  ( -25.99999999999999645, 9.999999999999994671, -7.500000000000000000 ) ) ;
#15899=EDGE_CURVE ( 'NONE', #8072, #4749, #17501, .T. ) ;
#15903=CARTESIAN_POINT ( 'NONE',  ( 0.000000000000000000, 0.000000000000000000, 0.000000000000000000 ) ) ;
#15911=CARTESIAN_POINT ( 'NONE',  ( -31.81644051279125662, 65.48968590022897729, 2.492004793192827972 ) ) ;
#15919=CIRCLE ( 'NONE', #12871, 4.999999999999995559 ) ;
#15922=CARTESIAN_POINT ( 'NONE',  ( -3.132434197188862957, 70.94952981831174554, 1.317303739528327577 ) ) ;
#15924=EDGE_CURVE ( 'NONE', #9496, #4124, #13760, .T. ) ;
#15929=DIRECTION ( 'NONE',  ( -0.000000000000000000, 1.000000000000000000, -0.000000000000000000 ) ) ;
#15930=ORIENTED_EDGE ( 'NONE', *, *, #18722, .F. ) ;
#15943=VECTOR ( 'NONE', #5870, 1000.000000000000000 ) ;
#15945=CARTESIAN_POINT ( 'NONE',  ( -15.99999999999999289, 65.74999999999998579, 4.999999999999989342 ) ) ;
#15947=CARTESIAN_POINT ( 'NONE',  ( -15.99999999999999289, 0.000000000000000000, 0.000000000000000000 ) ) ;
#15975=VECTOR ( 'NONE', #6602, 1000.000000000000000 ) ;
#15985=CARTESIAN_POINT ( 'NONE',  ( 28.00000000000001066, 64.25000000000000000, -1.525597966175989972 ) ) ;
#15992=CARTESIAN_POINT ( 'NONE',  ( -10.36407271659200369, 45.24472543703319616, -11.16260780707907685 ) ) ;
#15994=AXIS2_PLACEMENT_3D ( 'NONE', #2916, #20494, #18816 ) ;
#16002=CARTESIAN_POINT ( 'NONE',  ( -4.047976277355980201, 79.14876326484314006, -7.307758369674530741 ) ) ;
#16005=ORIENTED_EDGE ( 'NONE', *, *, #3457, .T. ) ;
#16008=CARTESIAN_POINT ( 'NONE',  ( -32.72864378893952875, 57.92794788011308782, 0.7338665021735866212 ) ) ;
#16013=CARTESIAN_POINT ( 'NONE',  ( 1.078027122475627042, 73.66227117401368218, -0.2439945722892260527 ) ) ;
#16015=AXIS2_PLACEMENT_3D ( 'NONE', #18562, #10802, #20350 ) ;
#16024=CARTESIAN_POINT ( 'NONE',  ( -27.57431306967301765, 71.02946758568791097, 4.727326826884577393 ) ) ;
#16032=CARTESIAN_POINT ( 'NONE',  ( -2.019385899523460370, 64.25000000000001421, 2.827122728375884186 ) ) ;
#16035=CARTESIAN_POINT ( 'NONE',  ( -30.62802697534700869, 79.12678444398457600, -7.447389982869642822 ) ) ;
#16040=DIRECTION ( 'NONE',  ( -0.000000000000000000, 1.000000000000000000, -0.000000000000000000 ) ) ;
#16042=DIRECTION ( 'NONE',  ( 1.000000000000000000, 0.000000000000000000, -0.000000000000000000 ) ) ;
#16057=CARTESIAN_POINT ( 'NONE',  ( -14.99999999999999645, 5.000000000000000000, 15.00000000000000000 ) ) ;
#16068=CARTESIAN_POINT ( 'NONE',  ( -29.44791497984978790, 77.20859777394102252, -3.699063880715452779 ) ) ;
#16085=CARTESIAN_POINT ( 'NONE',  ( -27.63707102110206293, 9.448329371371865903, -4.575993311049476375 ) ) ;
#16092=CARTESIAN_POINT ( 'NONE',  ( -9.429792107721615579, 50.26201249766958057, -15.29528091781460297 ) ) ;
#16098=ORIENTED_EDGE ( 'NONE', *, *, #2378, .T. ) ;
#16102=CARTESIAN_POINT ( 'NONE',  ( -3.402542903551478926, 78.78634076744670267, -6.409256716261817033 ) ) ;
#16107=CARTESIAN_POINT ( 'NONE',  ( -19.67995207262838520, 60.86351781624375690, -3.389291572743973635 ) ) ;
#16119=CARTESIAN_POINT ( 'NONE',  ( -27.74827478545477888, 57.32317209004575176, 4.280504417503601111 ) ) ;
#16122=DIRECTION ( 'NONE',  ( 0.000000000000000000, 1.000000000000000000, 0.000000000000000000 ) ) ;
#16123=DIRECTION ( 'NONE',  ( -0.000000000000000000, -1.000000000000000000, -0.000000000000000000 ) ) ;
#16128=EDGE_LOOP ( 'NONE', ( #13915, #9763, #2377, #14875 ) ) ;
#16136=ADVANCED_FACE ( 'NONE', ( #6089 ), #20312, .F. ) ;
#16138=CIRCLE ( 'NONE', #6972, 4.999999999999989342 ) ;
#16153=CARTESIAN_POINT ( 'NONE',  ( 10.49211908931699178, 0.000000000000000000, 0.000000000000000000 ) ) ;
#16155=CARTESIAN_POINT ( 'NONE',  ( -28.48915680482255652, 80.00000000000000000, 0.5205403966592361265 ) ) ;
#16160=ORIENTED_EDGE ( 'NONE', *, *, #10561, .F. ) ;
#16162=CARTESIAN_POINT ( 'NONE',  ( -31.96408918797520471, 67.75983095507351095, 2.252573492070595318 ) ) ;
#16182=PLANE ( 'NONE',  #1737 ) ;
#16185=DIRECTION ( 'NONE',  ( 0.000000000000000000, 0.000000000000000000, -1.000000000000000000 ) ) ;
#16186=ORIENTED_EDGE ( 'NONE', *, *, #14045, .F. ) ;
#16192=CARTESIAN_POINT ( 'NONE',  ( -0.2021197016317256845, 50.46427967968534034, -8.782110831005875085 ) ) ;
#16199=CARTESIAN_POINT ( 'NONE',  ( -13.40786934824189558, 79.99957779460261520, -12.37049764041790390 ) ) ;
#16212=DIRECTION ( 'NONE',  ( -0.000000000000000000, -1.000000000000000000, -0.000000000000000000 ) ) ;
#16220=AXIS2_PLACEMENT_3D ( 'NONE', #17515, #9433, #16042 ) ;
#16224=ORIENTED_EDGE ( 'NONE', *, *, #4691, .F. ) ;
#16250=FACE_OUTER_BOUND ( 'NONE', #11218, .T. ) ;
#16262=CARTESIAN_POINT ( 'NONE',  ( -29.55307521651278435, 64.25000000000002842, 3.020008312198915412 ) ) ;
#16268=ORIENTED_EDGE ( 'NONE', *, *, #3457, .F. ) ;
#16281=AXIS2_PLACEMENT_3D ( 'NONE', #5293, #11679, #14679 ) ;
#16284=VECTOR ( 'NONE', #4793, 1000.000000000000000 ) ;
#16287=CARTESIAN_POINT ( 'NONE',  ( -4.681704537686387724, 62.69813775908227171, 5.305497683706574819 ) ) ;
#16292=CARTESIAN_POINT ( 'NONE',  ( -4.343379421876969460, 58.21999429253379077, 4.515609508575330722 ) ) ;
#16295=DIRECTION ( 'NONE',  ( -0.000000000000000000, -0.000000000000000000, 1.000000000000000000 ) ) ;
#16328=ORIENTED_EDGE ( 'NONE', *, *, #11344, .T. ) ;
#16330=EDGE_LOOP ( 'NONE', ( #4560, #14594, #1625, #15555 ) ) ;
#16339=FACE_OUTER_BOUND ( 'NONE', #11568, .T. ) ;
#16349=AXIS2_PLACEMENT_3D ( 'NONE', #3857, #682, #18176 ) ;
#16352=ORIENTED_EDGE ( 'NONE', *, *, #162, .F. ) ;
#16353=DIRECTION ( 'NONE',  ( 0.000000000000000000, 0.000000000000000000, 1.000000000000000000 ) ) ;
#16357=ORIENTED_EDGE ( 'NONE', *, *, #17815, .T. ) ;
#16359=ADVANCED_FACE ( 'NONE', ( #3641 ), #907, .F. ) ;
#16360=VERTEX_POINT ( 'NONE', #10306 ) ;
#16365=ORIENTED_EDGE ( 'NONE', *, *, #14210, .T. ) ;
#16369=DIRECTION ( 'NONE',  ( 0.000000000000000000, 1.000000000000000000, 0.000000000000000000 ) ) ;
#16372=ORIENTED_EDGE ( 'NONE', *, *, #8756, .T. ) ;
#16374=AXIS2_PLACEMENT_3D ( 'NONE', #9334, #15244, #13530 ) ;
#16386=CARTESIAN_POINT ( 'NONE',  ( -26.20384780446736173, 9.999999997039491717, -7.228202927376838893 ) ) ;
#16387=CIRCLE ( 'NONE', #19746, 4.999999999999999112 ) ;
#16393=CARTESIAN_POINT ( 'NONE',  ( -3.848310109324514006, 46.83026313486608672, -2.948019393338978222 ) ) ;
#16396=CARTESIAN_POINT ( 'NONE',  ( -3.651764899804558429, 52.03701157797662091, 1.955602390459402873 ) ) ;
#16401=ORIENTED_EDGE ( 'NONE', *, *, #675, .F. ) ;
#16406=CARTESIAN_POINT ( 'NONE',  ( -15.99999999999999289, -9.999999999999994671, 0.000000000000000000 ) ) ;
#16412=CARTESIAN_POINT ( 'NONE',  ( -13.69112006203626564, 59.06815658944699976, -4.446547635559181977 ) ) ;
#16422=CARTESIAN_POINT ( 'NONE',  ( -28.28208682648537220, 52.78748761784272148, -3.776222344276643827 ) ) ;
#16424=EDGE_CURVE ( 'NONE', #6609, #8072, #19535, .T. ) ;
#16448=CARTESIAN_POINT ( 'NONE',  ( -15.99999999999991651, 71.61437827766162911, -4.999999999999997335 ) ) ;
#16452=ORIENTED_EDGE ( 'NONE', *, *, #11471, .F. ) ;
#16453=AXIS2_PLACEMENT_3D ( 'NONE', #20732, #10559, #15467 ) ;
#16460=CARTESIAN_POINT ( 'NONE',  ( -19.61372346390630028, 79.99792423946925624, -12.24236967450913660 ) ) ;
#16472=DIRECTION ( 'NONE',  ( 0.7999999999999998224, 0.000000000000000000, -0.6000000000000000888 ) ) ;
#16474=CYLINDRICAL_SURFACE ( 'NONE', #49, 15.00000000000000000 ) ;
#16482=CARTESIAN_POINT ( 'NONE',  ( -27.93151244679091505, 6.473849509709803662, -3.824115908589273971 ) ) ;
#16492=CARTESIAN_POINT ( 'NONE',  ( -3.221035240742360362, 54.22335479770934086, -2.040458165079695796 ) ) ;
#16493=CARTESIAN_POINT ( 'NONE',  ( -15.53444873921510272, 80.00000000000001421, -12.49812590152206404 ) ) ;
#16503=VERTEX_POINT ( 'NONE', #17721 ) ;
#16508=CARTESIAN_POINT ( 'NONE',  ( -16.18042569387133511, 58.38562172233856984, -4.999999999999989342 ) ) ;
#16514=CARTESIAN_POINT ( 'NONE',  ( 0.000000000000000000, -10.00000000000000000, 0.000000000000000000 ) ) ;
#16522=CARTESIAN_POINT ( 'NONE',  ( -28.94626959558488011, 56.84162378296022666, 0.1050044003684389854 ) ) ;
#16523=CARTESIAN_POINT ( 'NONE',  ( -16.32953223445319679, 20.09941697557067997, 12.50000000000000178 ) ) ;
#16526=( BOUNDED_SURFACE ( )  B_SPLINE_SURFACE ( 3, 2, ( 
 ( #13897, #4248, #13796 ),
 ( #12202, #16864, #2345 ),
 ( #8803, #9103, #8695 ),
 ( #15302, #18775, #20143 ),
 ( #5606, #10699, #19927 ),
 ( #12094, #5394, #20245 ),
 ( #18563, #18351, #4143 ),
 ( #10481, #17081, #16758 ),
 ( #7307, #2240, #2453 ),
 ( #15404, #2560, #9005 ),
 ( #16024, #7730, #20456 ),
 ( #15715, #19289, #20862 ),
 ( #6336, #20558, #6136 ),
 ( #1486, #4759, #2769 ),
 ( #3176, #10803, #17283 ),
 ( #11241, #1285, #15911 ) ),
 .UNSPECIFIED., .F., .F., .T. ) 
 B_SPLINE_SURFACE_WITH_KNOTS ( ( 4, 2, 2, 2, 2, 2, 2, 4 ),
 ( 3, 3 ),
 ( 0.09394529277310080528, 0.09803747693844724886, 0.1000835690211204776, 0.1011066150624570781, 0.1021296611037936924, 0.1062218452691401360, 0.1082679373518133648, 0.1103140294344865796 ),
 ( 0.000000000000000000, 1.000000000000000000 ),
 .UNSPECIFIED. ) 
 GEOMETRIC_REPRESENTATION_ITEM ( )  RATIONAL_B_SPLINE_SURFACE ( (
 ( 1.000000000000000000, 0.7167790485004653656, 1.000000000000000000),
 ( 1.000000000000000000, 0.7312157917998166612, 1.000000000000000000),
 ( 1.000000000000000000, 0.7466500244729707969, 1.000000000000000000),
 ( 1.000000000000000000, 0.7689011243010751562, 1.000000000000000000),
 ( 1.000000000000000000, 0.7761748643738399789, 1.000000000000000000),
 ( 1.000000000000000000, 0.7866334538989935288, 1.000000000000000000),
 ( 1.000000000000000000, 0.7900487569768197549, 1.000000000000000000),
 ( 1.000000000000000000, 0.7966228133242926335, 1.000000000000000000),
 ( 1.000000000000000000, 0.7997907721098268530, 1.000000000000000000),
 ( 1.000000000000000000, 0.8149753752735824364, 1.000000000000000000),
 ( 1.000000000000000000, 0.8250225257833745385, 1.000000000000000000),
 ( 1.000000000000000000, 0.8359195949012849791, 1.000000000000000000),
 ( 1.000000000000000000, 0.8388534816487658308, 1.000000000000000000),
 ( 1.000000000000000000, 0.8430760250471756034, 1.000000000000000000),
 ( 1.000000000000000000, 0.8443918141125164034, 1.000000000000000000),
 ( 1.000000000000000000, 0.8449065510952332714, 1.000000000000000000) ) ) 
 REPRESENTATION_ITEM ( '' )  SURFACE ( )  );
#16527=VERTEX_POINT ( 'NONE', #19596 ) ;
#16530=ORIENTED_EDGE ( 'NONE', *, *, #6831, .T. ) ;
#16541=CARTESIAN_POINT ( 'NONE',  ( -29.34053455105015829, 65.74999999999997158, 3.134647201270610140 ) ) ;
#16557=CARTESIAN_POINT ( 'NONE',  ( -12.00682109638796291, 68.17699921526258322, -3.011576861204072753 ) ) ;
#16565=ORIENTED_EDGE ( 'NONE', *, *, #3336, .T. ) ;
#16567=CARTESIAN_POINT ( 'NONE',  ( -19.56641610727023561, 79.99999999999583622, -11.99131545410286925 ) ) ;
#16572=VECTOR ( 'NONE', #4492, 1000.000000000000000 ) ;
#16575=ORIENTED_EDGE ( 'NONE', *, *, #8792, .T. ) ;
#16579=CARTESIAN_POINT ( 'NONE',  ( -13.42396981071245854, 80.00000000000414957, -12.24234612424543478 ) ) ;
#16581=AXIS2_PLACEMENT_3D ( 'NONE', #8748, #4088, #5555 ) ;
#16587=CARTESIAN_POINT ( 'NONE',  ( -28.49991287530916040, 6.470303912909706412, -0.3949351193324712184 ) ) ;
#16592=CARTESIAN_POINT ( 'NONE',  ( -6.481806088851808312, 45.01191145235649316, -8.139083654344593910 ) ) ;
#16596=CARTESIAN_POINT ( 'NONE',  ( -3.688831311464842777, 52.40708535496389686, 2.175092931272005981 ) ) ;
#16615=EDGE_CURVE ( 'NONE', #12912, #6578, #11063, .T. ) ;
#16619=CYLINDRICAL_SURFACE ( 'NONE', #18538, 4.999999999999989342 ) ;
#16624=CARTESIAN_POINT ( 'NONE',  ( -27.91715957486725230, 46.29657224408730798, -3.824975988489407897 ) ) ;
#16626=AXIS2_PLACEMENT_3D ( 'NONE', #13437, #11738, #5247 ) ;
#16637=ORIENTED_EDGE ( 'NONE', *, *, #6523, .F. ) ;
#16652=CARTESIAN_POINT ( 'NONE',  ( 1.484819526751607999, 80.00000000000000000, 0.7287565553229443660 ) ) ;
#16653=DIRECTION ( 'NONE',  ( 0.000000000000000000, 0.000000000000000000, -1.000000000000000000 ) ) ;
#16662=CONICAL_SURFACE ( 'NONE', #15994, 4.999999999999995559, 1.029744258676653867 ) ;
#16665=CARTESIAN_POINT ( 'NONE',  ( -13.09058959453371074, 70.37881519986052581, -4.068652614656581790 ) ) ;
#16674=CARTESIAN_POINT ( 'NONE',  ( -17.30218132643816276, 79.99997331865614569, -12.46740305798945592 ) ) ;
#16692=CARTESIAN_POINT ( 'NONE',  ( -0.4956845319646441261, 78.79719334215242554, -6.605250029488230368 ) ) ;
#16701=CARTESIAN_POINT ( 'NONE',  ( -29.99999999999999645, 5.000000000000000000, 8.929304381912043453 ) ) ;
#16706=CARTESIAN_POINT ( 'NONE',  ( -8.767231887450829930, 45.07424775628126667, -10.22364500895912798 ) ) ;
#16710=CARTESIAN_POINT ( 'NONE',  ( -3.063870802415169070, 57.44566917294824293, 0.4923802658666992516 ) ) ;
#16711=CARTESIAN_POINT ( 'NONE',  ( -1.372481614566710251, 79.12694522062832903, -7.447838812965425603 ) ) ;
#16728=DIRECTION ( 'NONE',  ( 6.608470384673549052E-16, -1.000000000000000000, 0.000000000000000000 ) ) ;
#16729=CARTESIAN_POINT ( 'NONE',  ( -15.99999999999991651, 71.61437827766162911, -4.999999999999997335 ) ) ;
#16731=CARTESIAN_POINT ( 'NONE',  ( -15.99999999999999289, 80.00000000000000000, 0.000000000000000000 ) ) ;
#16732=CARTESIAN_POINT ( 'NONE',  ( -26.65066008881222359, 45.27454425555390571, -6.552074931230112753 ) ) ;
#16738=ORIENTED_EDGE ( 'NONE', *, *, #6930, .T. ) ;
#16743=DIRECTION ( 'NONE',  ( 1.000000000000000000, 0.000000000000000000, 0.000000000000000000 ) ) ;
#16749=CARTESIAN_POINT ( 'NONE',  ( 10.49211908931699178, 5.000000000000000000, -5.000000000000000000 ) ) ;
#16758=CARTESIAN_POINT ( 'NONE',  ( -32.68029730050665194, 71.85025536417415992, 0.8468720397201384698 ) ) ;
#16772=DIRECTION ( 'NONE',  ( 0.000000000000000000, 0.000000000000000000, -1.000000000000000000 ) ) ;
#16785=CARTESIAN_POINT ( 'NONE',  ( -11.09026189855725164, 15.09941697557061957, 0.9457651797582804498 ) ) ;
#16786=ORIENTED_EDGE ( 'NONE', *, *, #5205, .F. ) ;
#16789=AXIS2_PLACEMENT_3D ( 'NONE', #3341, #9478, #17672 ) ;
#16801=DIRECTION ( 'NONE',  ( 1.000000000000000000, 0.000000000000000000, 0.000000000000000000 ) ) ;
#16802=CARTESIAN_POINT ( 'NONE',  ( -35.00000000000000000, 65.00000000000000000, -12.50000000000000000 ) ) ;
#16814=EDGE_CURVE ( 'NONE', #11795, #7840, #15837, .T. ) ;
#16832=CIRCLE ( 'NONE', #7676, 4.999999999999993783 ) ;
#16835=CARTESIAN_POINT ( 'NONE',  ( -25.80684929261252236, 50.42143158553669480, -7.768010691411298296 ) ) ;
#16842=EDGE_LOOP ( 'NONE', ( #6149, #10113 ) ) ;
#16855=DIRECTION ( 'NONE',  ( 0.000000000000000000, 0.000000000000000000, -1.000000000000000000 ) ) ;
#16860=DIRECTION ( 'NONE',  ( 0.000000000000000000, 0.000000000000000000, -1.000000000000000000 ) ) ;
#16863=ORIENTED_EDGE ( 'NONE', *, *, #12522, .T. ) ;
#16864=CARTESIAN_POINT ( 'NONE',  ( -28.78409816537090293, 75.81673797948198512, -2.071606702223387941 ) ) ;
#16868=EDGE_CURVE ( 'NONE', #2271, #16360, #20513, .T. ) ;
#16871=CONICAL_SURFACE ( 'NONE', #2319, 9.999999999999998224, 0.7853981633974561616 ) ;
#16873=CARTESIAN_POINT ( 'NONE',  ( -15.99999999999999289, 65.74999999999998579, 0.000000000000000000 ) ) ;
#16881=CARTESIAN_POINT ( 'NONE',  ( -16.52214123053562744, 80.00000332749893062, -12.49385289755934991 ) ) ;
#16882=DIRECTION ( 'NONE',  ( -1.000000000000000000, 0.000000000000000000, -0.000000000000000000 ) ) ;
#16903=DIRECTION ( 'NONE',  ( -0.000000000000000000, 1.000000000000000000, -0.000000000000000000 ) ) ;
#16911=ORIENTED_EDGE ( 'NONE', *, *, #9247, .F. ) ;
#16918=ORIENTED_EDGE ( 'NONE', *, *, #11349, .F. ) ;
#16926=DIRECTION ( 'NONE',  ( 0.000000000000000000, 0.000000000000000000, -1.000000000000000000 ) ) ;
#16935=EDGE_CURVE ( 'NONE', #4880, #17792, #3974, .T. ) ;
#16937=CARTESIAN_POINT ( 'NONE',  ( -23.58898520603824167, 49.74445733756040511, -9.939908570437406610 ) ) ;
#16951=CARTESIAN_POINT ( 'NONE',  ( 0.000000000000000000, 5.000000000000000000, 0.000000000000000000 ) ) ;
#16966=CARTESIAN_POINT ( 'NONE',  ( -12.23590939273504041, 18.40648074834063053, 11.92219499127797810 ) ) ;
#16975=ORIENTED_EDGE ( 'NONE', *, *, #19951, .F. ) ;
#16989=DIRECTION ( 'NONE',  ( -0.000000000000000000, -0.000000000000000000, 1.000000000000000000 ) ) ;
#17002=CARTESIAN_POINT ( 'NONE',  ( -35.00000000000000000, 65.74999999999997158, 75.00000000000000000 ) ) ;
#17009=CARTESIAN_POINT ( 'NONE',  ( -11.03318111385504707, 14.43719822709678802, 11.47107871140386415 ) ) ;
#17015=CARTESIAN_POINT ( 'NONE',  ( -29.99999999999999645, 4.999999999999999112, -1.892809692664370491 ) ) ;
#17024=CARTESIAN_POINT ( 'NONE',  ( -0.1835734997365038312, 64.12228024131808013, 2.492032687065257601 ) ) ;
#17035=CARTESIAN_POINT ( 'NONE',  ( -28.48915680482256008, 80.00000000000000000, 0.5205403966592370146 ) ) ;
#17045=CARTESIAN_POINT ( 'NONE',  ( -19.21593171750998863, 70.00183809964329384, -3.834978693179198928 ) ) ;
#17047=DIRECTION ( 'NONE',  ( 0.7071067811865420216, 0.000000000000000000, -0.7071067811865531239 ) ) ;
#17050=CARTESIAN_POINT ( 'NONE',  ( -13.26898700413883958, 45.53651568644503556, -12.21732978123357505 ) ) ;
#17051=DIRECTION ( 'NONE',  ( -1.000000000000000000, -0.000000000000000000, -0.000000000000000000 ) ) ;
#17054=CARTESIAN_POINT ( 'NONE',  ( -27.33357274664675884, 62.70188032564514913, 5.273416595308242805 ) ) ;
#17055=ORIENTED_EDGE ( 'NONE', *, *, #5054, .T. ) ;
#17066=CARTESIAN_POINT ( 'NONE',  ( 1.494606444039509041, 52.93669486463471685, -3.576234255370625448 ) ) ;
#17067=CARTESIAN_POINT ( 'NONE',  ( -46.99999999999998579, 65.74999999999995737, -2.528164662410434804 ) ) ;
#17077=ADVANCED_FACE ( 'NONE', ( #19469 ), #16619, .F. ) ;
#17081=CARTESIAN_POINT ( 'NONE',  ( -28.92569456491105484, 72.33610889978091052, 0.5975377147109768305 ) ) ;
#17094=CARTESIAN_POINT ( 'NONE',  ( -29.99999999999999645, 9.999999999999994671, -10.49999999999999822 ) ) ;
#17098=CARTESIAN_POINT ( 'NONE',  ( -15.99999999999999289, 15.09941697557068530, 15.00000000000000000 ) ) ;
#17106=DIRECTION ( 'NONE',  ( 0.8571673007021120005, 0.000000000000000000, 0.5150380749100547106 ) ) ;
#17112=CARTESIAN_POINT ( 'NONE',  ( -11.00000000000000355, 14.76511876738014628, 11.45643923738960623 ) ) ;
#17114=VECTOR ( 'NONE', #408, 1000.000000000000000 ) ;
#17121=FACE_OUTER_BOUND ( 'NONE', #6260, .T. ) ;
#17138=CARTESIAN_POINT ( 'NONE',  ( -19.76842508384192598, 11.79734777244101984, 11.92081118759508129 ) ) ;
#17150=CARTESIAN_POINT ( 'NONE',  ( -16.75433277476891547, 49.50806098447029058, -12.49936755495519414 ) ) ;
#17151=DIRECTION ( 'NONE',  ( 0.000000000000000000, 0.000000000000000000, -1.000000000000000000 ) ) ;
#17153=CARTESIAN_POINT ( 'NONE',  ( -28.46671850446983854, 50.53532148300114102, 0.9425010236277686637 ) ) ;
#17156=EDGE_LOOP ( 'NONE', ( #20658, #13766, #3744, #3414 ) ) ;
#17165=CARTESIAN_POINT ( 'NONE',  ( -5.474186428702649820, 50.03685501615670006, -13.63068399189310931 ) ) ;
#17166=DIRECTION ( 'NONE',  ( -1.000000000000000000, 0.000000000000000000, 0.000000000000000000 ) ) ;
#17179=EDGE_CURVE ( 'NONE', #9209, #13744, #3808, .T. ) ;
#17183=CARTESIAN_POINT ( 'NONE',  ( -11.10102051443364779, 14.09941697557065332, 0.9999999999999991118 ) ) ;
#17196=CARTESIAN_POINT ( 'NONE',  ( -35.00000000000000000, 65.00000000000000000, -12.50000000000000000 ) ) ;
#17199=DIRECTION ( 'NONE',  ( 0.000000000000000000, 0.000000000000000000, -1.000000000000000000 ) ) ;
#17200=CARTESIAN_POINT ( 'NONE',  ( 1.484819526751601559, 76.25000000000000000, -2.578432583507792142 ) ) ;
#17205=DIRECTION ( 'NONE',  ( 1.000000000000000000, 6.608470384673549052E-16, 0.000000000000000000 ) ) ;
#17211=CARTESIAN_POINT ( 'NONE',  ( -15.99999999999999289, 79.99999999999998579, -12.50000000000000178 ) ) ;
#17219=DIRECTION ( 'NONE',  ( 0.000000000000000000, 0.000000000000000000, 1.000000000000000000 ) ) ;
#17222=ORIENTED_EDGE ( 'NONE', *, *, #17421, .F. ) ;
#17228=DIRECTION ( 'NONE',  ( 0.000000000000000000, 0.000000000000000000, 1.000000000000000000 ) ) ;
#17236=ORIENTED_EDGE ( 'NONE', *, *, #9979, .F. ) ;
#17240=CARTESIAN_POINT ( 'NONE',  ( -20.33466442860505197, 12.58620624673167221, 11.72593040804455278 ) ) ;
#17244=CARTESIAN_POINT ( 'NONE',  ( 44.00000000000000000, 0.000000000000000000, 15.00000000000000000 ) ) ;
#17250=CARTESIAN_POINT ( 'NONE',  ( -19.35604988386060299, 50.41666730312486777, -16.01143037413084969 ) ) ;
#17254=CARTESIAN_POINT ( 'NONE',  ( -27.46410040126770724, 60.39801160101181665, 4.985054410776884382 ) ) ;
#17256=EDGE_LOOP ( 'NONE', ( #18102, #626, #11793, #7971, #13605, #17426, #6668, #13229, #17055, #7999, #345, #16005, #18101, #19486, #353, #11383 ) ) ;
#17261=CARTESIAN_POINT ( 'NONE',  ( -3.499198184780732745, 80.00000000000000000, 0.2411454413945828268 ) ) ;
#17265=DIRECTION ( 'NONE',  ( 0.000000000000000000, 1.000000000000000000, 0.000000000000000000 ) ) ;
#17267=CARTESIAN_POINT ( 'NONE',  ( -26.56874857031798598, 50.03503563072523974, -13.60624899383130071 ) ) ;
#17269=VERTEX_POINT ( 'NONE', #17244 ) ;
#17283=CARTESIAN_POINT ( 'NONE',  ( -31.82693145428951098, 65.99841087575286736, 2.475388239833567372 ) ) ;
#17285=CARTESIAN_POINT ( 'NONE',  ( 27.00000000000002487, 65.00000000000000000, -27.49999999999999645 ) ) ;
#17292=EDGE_CURVE ( 'NONE', #6578, #491, #5988, .T. ) ;
#17293=ORIENTED_EDGE ( 'NONE', *, *, #20128, .F. ) ;
#17302=PLANE ( 'NONE',  #14514 ) ;
#17304=CARTESIAN_POINT ( 'NONE',  ( 10.49211908931699178, -10.00000000000000000, -5.999999999999998224 ) ) ;
#17313=CYLINDRICAL_SURFACE ( 'NONE', #14853, 5.999999999999989342 ) ;
#17314=EDGE_LOOP ( 'NONE', ( #20203, #14807, #19132, #14958 ) ) ;
#17320=CARTESIAN_POINT ( 'NONE',  ( -28.96704929677014917, 76.49637892406967410, -2.857129581998074208 ) ) ;
#17332=AXIS2_PLACEMENT_3D ( 'NONE', #13725, #5323, #11814 ) ;
#17334=ORIENTED_EDGE ( 'NONE', *, *, #10976, .F. ) ;
#17339=CARTESIAN_POINT ( 'NONE',  ( 30.10683012259193703, 0.000000000000000000, 0.000000000000000000 ) ) ;
#17342=LINE ( 'NONE', #19039, #17622 ) ;
#17344=VERTEX_POINT ( 'NONE', #15985 ) ;
#17349=CIRCLE ( 'NONE', #12268, 13.99999999999999822 ) ;
#17354=CARTESIAN_POINT ( 'NONE',  ( -46.99999999999998579, 65.74999999999995737, -2.528164662410434804 ) ) ;
#17364=CARTESIAN_POINT ( 'NONE',  ( -18.39717848847821813, 45.55555640428114828, -12.27279083252108016 ) ) ;
#17371=CYLINDRICAL_SURFACE ( 'NONE', #11542, 14.99999999999999645 ) ;
#17373=CARTESIAN_POINT ( 'NONE',  ( 1.320351081125068049, 77.22491497699002139, -3.799191488835419683 ) ) ;
#17378=CARTESIAN_POINT ( 'NONE',  ( 1.332880925387092796, 55.04869403453741938, -1.249173068972419198 ) ) ;
#17379=CARTESIAN_POINT ( 'NONE',  ( -28.99999999999999289, 0.000000000000000000, 15.00000000000000178 ) ) ;
#17400=CARTESIAN_POINT ( 'NONE',  ( -4.085501928355141033, 74.13367381892273045, 3.782735275915807716 ) ) ;
#17410=CARTESIAN_POINT ( 'NONE',  ( -11.09026189855742572, 14.76386108487820259, 0.9457651797581829722 ) ) ;
#17413=CARTESIAN_POINT ( 'NONE',  ( 28.00000000000001066, 65.75000000000001421, 75.00000000000000000 ) ) ;
#17417=DIRECTION ( 'NONE',  ( -0.000000000000000000, -1.000000000000000000, -0.000000000000000000 ) ) ;
#17421=EDGE_CURVE ( 'NONE', #14829, #10630, #8023, .T. ) ;
#17424=CARTESIAN_POINT ( 'NONE',  ( -20.89897948556633978, 14.09941697557065332, 0.9999999999999991118 ) ) ;
#17426=ORIENTED_EDGE ( 'NONE', *, *, #20480, .T. ) ;
#17431=ADVANCED_FACE ( 'NONE', ( #8203 ), #14812, .F. ) ;
#17434=DIRECTION ( 'NONE',  ( -0.000000000000000000, 1.000000000000000000, -0.000000000000000000 ) ) ;
#17437=EDGE_CURVE ( 'NONE', #166, #1421, #11773, .T. ) ;
#17443=FACE_OUTER_BOUND ( 'NONE', #11313, .T. ) ;
#17446=ORIENTED_EDGE ( 'NONE', *, *, #13273, .F. ) ;
#17453=DIRECTION ( 'NONE',  ( 0.000000000000000000, 0.000000000000000000, 1.000000000000000000 ) ) ;
#17463=CIRCLE ( 'NONE', #19154, 13.99999999999999822 ) ;
#17465=CARTESIAN_POINT ( 'NONE',  ( 0.6679515277691319142, 50.95756615319989891, -7.179599708890708420 ) ) ;
#17470=CARTESIAN_POINT ( 'NONE',  ( -26.84899328648689476, 45.33011328186441347, -6.253688604731005185 ) ) ;
#17472=EDGE_LOOP ( 'NONE', ( #15114, #7195, #18135, #6443 ) ) ;
#17481=CARTESIAN_POINT ( 'NONE',  ( -10.57486132309840521, 50.32666072867165497, -15.61762382048297404 ) ) ;
#17485=ORIENTED_EDGE ( 'NONE', *, *, #9772, .F. ) ;
#17487=CARTESIAN_POINT ( 'NONE',  ( -0.1767699604045824824, 65.74999999999997158, 2.481238266578629226 ) ) ;
#17494=CARTESIAN_POINT ( 'NONE',  ( -28.65135327001111065, 64.04126923566909113, 2.490177094220571430 ) ) ;
#17500=CARTESIAN_POINT ( 'NONE',  ( -15.99999999999999289, 80.00000000000000000, 0.000000000000000000 ) ) ;
#17501=CIRCLE ( 'NONE', #12078, 12.50000000000000000 ) ;
#17507=CARTESIAN_POINT ( 'NONE',  ( -28.99999999999999289, -10.00000000000000000, 15.00000000000000178 ) ) ;
#17508=EDGE_CURVE ( 'NONE', #18381, #3402, #10847, .T. ) ;
#17515=CARTESIAN_POINT ( 'NONE',  ( 30.00000000000000000, 0.000000000000000000, 28.99999999999999645 ) ) ;
#17522=CARTESIAN_POINT ( 'NONE',  ( -14.99999999999999645, -10.00000000000000000, -28.99999999999999645 ) ) ;
#17538=CARTESIAN_POINT ( 'NONE',  ( -27.87293505806218619, 79.99999999978210496, -3.927153389733302191 ) ) ;
#17545=VERTEX_POINT ( 'NONE', #10965 ) ;
#17548=EDGE_CURVE ( 'NONE', #8656, #681, #7349, .T. ) ;
#17564=ORIENTED_EDGE ( 'NONE', *, *, #12522, .F. ) ;
#17570=CARTESIAN_POINT ( 'NONE',  ( -6.040070365067144564, 50.06279613334914558, -13.94107049437905665 ) ) ;
#17571=DIRECTION ( 'NONE',  ( 0.000000000000000000, -1.000000000000000000, 0.000000000000000000 ) ) ;
#17574=CARTESIAN_POINT ( 'NONE',  ( -15.99999999999998934, 45.63508326896292289, -12.50000000000000000 ) ) ;
#17576=VERTEX_POINT ( 'NONE', #5105 ) ;
#17580=ORIENTED_EDGE ( 'NONE', *, *, #19118, .F. ) ;
#17589=ORIENTED_EDGE ( 'NONE', *, *, #1655, .F. ) ;
#17597=CARTESIAN_POINT ( 'NONE',  ( -31.81189201763190511, 64.84542049530487873, 2.499203484743047099 ) ) ;
#17611=CARTESIAN_POINT ( 'NONE',  ( 1.484819526751601559, 76.25000000000000000, -2.578432583507792586 ) ) ;
#17619=FACE_OUTER_BOUND ( 'NONE', #1947, .T. ) ;
#17622=VECTOR ( 'NONE', #4196, 1000.000000000000000 ) ;
#17624=LINE ( 'NONE', #3300, #9214 ) ;
#17628=DIRECTION ( 'NONE',  ( 0.000000000000000000, 0.000000000000000000, -1.000000000000000000 ) ) ;
#17644=ORIENTED_EDGE ( 'NONE', *, *, #8234, .F. ) ;
#17647=CARTESIAN_POINT ( 'NONE',  ( -29.18969730202500301, 79.49366880382837053, -8.593311550915920805 ) ) ;
#17664=CARTESIAN_POINT ( 'NONE',  ( 30.10683012259193703, -10.00000000000000000, 4.999999999999997335 ) ) ;
#17672=DIRECTION ( 'NONE',  ( 0.000000000000000000, 0.000000000000000000, 1.000000000000000000 ) ) ;
#17678=CARTESIAN_POINT ( 'NONE',  ( 1.114207876027680122, 51.53275387072061875, -5.884738422014940795 ) ) ;
#17683=CARTESIAN_POINT ( 'NONE',  ( -17.53792359058950723, 45.60860274098917699, -12.42895697958611123 ) ) ;
#17689=CARTESIAN_POINT ( 'NONE',  ( -4.382345773779359632, 80.00000000021817925, -4.628091497300713009 ) ) ;
#17692=CARTESIAN_POINT ( 'NONE',  ( -16.00000000000007105, 58.38562172233837089, -4.999999999999997335 ) ) ;
#17699=AXIS2_PLACEMENT_3D ( 'NONE', #13505, #12118, #19950 ) ;
#17704=CARTESIAN_POINT ( 'NONE',  ( -11.00000000000000355, 15.43320684789191333, 11.45643923738960446 ) ) ;
#17705=EDGE_CURVE ( 'NONE', #17269, #9496, #15624, .T. ) ;
#17707=CARTESIAN_POINT ( 'NONE',  ( -31.95547536107751796, 62.33962363497189330, 2.266630807618284393 ) ) ;
#17710=DIRECTION ( 'NONE',  ( 1.000000000000000000, -0.000000000000000000, -0.000000000000000000 ) ) ;
#17711=LINE ( 'NONE', #4762, #1062 ) ;
#17719=CARTESIAN_POINT ( 'NONE',  ( 0.9726465904711251165, 73.17878816827938238, 0.08443632836958642196 ) ) ;
#17721=CARTESIAN_POINT ( 'NONE',  ( 10.49211908931699178, 5.000000000000000000, 5.000000000000000000 ) ) ;
#17723=ADVANCED_FACE ( 'NONE', ( #5937 ), #18788, .F. ) ;
#17728=CIRCLE ( 'NONE', #16374, 5.000000000000000000 ) ;
#17734=ADVANCED_FACE ( 'NONE', ( #7643 ), #17302, .F. ) ;
#17748=ORIENTED_EDGE ( 'NONE', *, *, #18084, .T. ) ;
#17751=CARTESIAN_POINT ( 'NONE',  ( -27.18818224385167426, 79.75568800831801752, -9.793444445059897419 ) ) ;
#17756=DIRECTION ( 'NONE',  ( 0.000000000000000000, 0.000000000000000000, -1.000000000000000000 ) ) ;
#17757=FACE_OUTER_BOUND ( 'NONE', #11703, .T. ) ;
#17769=CARTESIAN_POINT ( 'NONE',  ( -26.92128470956473407, 9.836181565225405876, -6.090021476509787313 ) ) ;
#17773=CARTESIAN_POINT ( 'NONE',  ( -7.945426057903055117, 49.82671907149163815, -9.565339651835223833 ) ) ;
#17777=CARTESIAN_POINT ( 'NONE',  ( -22.91475887178305015, 45.10727738977845291, -10.42048756752374672 ) ) ;
#17778=VECTOR ( 'NONE', #5413, 1000.000000000000000 ) ;
#17780=VERTEX_POINT ( 'NONE', #12644 ) ;
#17782=CARTESIAN_POINT ( 'NONE',  ( 30.10683012259193703, 5.000000000000000000, -4.999999999999997335 ) ) ;
#17784=CARTESIAN_POINT ( 'NONE',  ( -6.621265648680998872, 79.74334935822896853, -9.599827418917257660 ) ) ;
#17792=VERTEX_POINT ( 'NONE', #5838 ) ;
#17796=DIRECTION ( 'NONE',  ( -0.000000000000000000, 1.000000000000000000, -0.000000000000000000 ) ) ;
#17798=CONICAL_SURFACE ( 'NONE', #533, 4.999999999999995559, 1.029744258676653867 ) ;
#17801=CARTESIAN_POINT ( 'NONE',  ( -32.14365289034154927, 60.93336360728059731, 1.942657716202586426 ) ) ;
#17815=EDGE_CURVE ( 'NONE', #10630, #14829, #14863, .T. ) ;
#17825=CARTESIAN_POINT ( 'NONE',  ( -31.82323003959540486, 64.25000000000000000, 2.481238266578627449 ) ) ;
#17828=EDGE_CURVE ( 'NONE', #3383, #12912, #1402, .T. ) ;
#17829=ADVANCED_FACE ( 'NONE', ( #9542 ), #4779, .F. ) ;
#17844=CARTESIAN_POINT ( 'NONE',  ( -13.69349610383069304, 70.93315970589998187, -4.447567583327517227 ) ) ;
#17847=VERTEX_POINT ( 'NONE', #3049 ) ;
#17850=UNCERTAINTY_MEASURE_WITH_UNIT (LENGTH_MEASURE( 1.000000000000000082E-05 ), #19126, 'distance_accuracy_value', 'NONE');
#17853=CARTESIAN_POINT ( 'NONE',  ( -32.98901474369844067, 73.25359183295174148, 0.03495786392106590285 ) ) ;
#17856=CARTESIAN_POINT ( 'NONE',  ( -32.97826049705485474, 77.74400922168739214, -4.586390192070082250 ) ) ;
#17871=CARTESIAN_POINT ( 'NONE',  ( 44.00000000000000000, -10.00000000000000000, 15.00000000000000000 ) ) ;
#17874=DIRECTION ( 'NONE',  ( 0.000000000000000000, 0.000000000000000000, -1.000000000000000000 ) ) ;
#17876=EDGE_CURVE ( 'NONE', #16527, #631, #19248, .T. ) ;
#17878=AXIS2_PLACEMENT_3D ( 'NONE', #9792, #1758, #16185 ) ;
#17884=CARTESIAN_POINT ( 'NONE',  ( -4.179710852470351234, 56.67225486372360876, 4.072319667107016983 ) ) ;
#17887=CARTESIAN_POINT ( 'NONE',  ( -8.109701803253319241, 50.18354407797716732, -14.84573819736936784 ) ) ;
#17888=CARTESIAN_POINT ( 'NONE',  ( -11.36219877386465882, 79.99567133403120067, -12.08300025664926558 ) ) ;
#17912=CARTESIAN_POINT ( 'NONE',  ( -27.32435382328680262, 62.88336031010526028, 5.293632132712875915 ) ) ;
#17914=ADVANCED_FACE ( 'NONE', ( #20330 ), #5417, .F. ) ;
#17923=CARTESIAN_POINT ( 'NONE',  ( -0.1835594872087454865, 65.48968590022838043, 2.492004793192846179 ) ) ;
#17935=B_SPLINE_CURVE_WITH_KNOTS ( 'NONE', 3,
 ( #20137, #7516, #4137, #5598, #8997, #851, #12087, #4023, #14007, #16966, #13788, #5702, #12194, #20450, #5916, #18871, #17704, #9410 ),
 .UNSPECIFIED., .F., .F.,
 ( 4, 2, 2, 2, 2, 2, 2, 2, 4 ),
 ( 0.02369296886942158509, 0.02467920192125608314, 0.02566543497309058119, 0.02665166802492507578, 0.02763790107675957383, 0.02862413412859407189, 0.02961036718042856647, 0.03059660023226306452, 0.03158283328409756258 ),
 .UNSPECIFIED. ) ;
#17951=ORIENTED_EDGE ( 'NONE', *, *, #20857, .F. ) ;
#17953=CARTESIAN_POINT ( 'NONE',  ( -15.99999999999999289, -10.00000000000000000, 0.000000000000000000 ) ) ;
#17968=AXIS2_PLACEMENT_3D ( 'NONE', #8888, #739, #16743 ) ;
#17973=DIRECTION ( 'NONE',  ( -0.000000000000000000, -1.000000000000000000, -0.000000000000000000 ) ) ;
#17985=CARTESIAN_POINT ( 'NONE',  ( -4.485171960567237548, 45.77964704178626221, -4.920232212067642941 ) ) ;
#17988=CARTESIAN_POINT ( 'NONE',  ( 0.3192688095861958009, 59.91499571937752933, 1.616389984123141721 ) ) ;
#18011=VECTOR ( 'NONE', #4245, 1000.000000000000000 ) ;
#18013=CARTESIAN_POINT ( 'NONE',  ( -28.31427895950539408, 52.41482254867882062, 2.195225357249351639 ) ) ;
#18018=ORIENTED_EDGE ( 'NONE', *, *, #11119, .F. ) ;
#18020=EDGE_LOOP ( 'NONE', ( #11841, #18018, #10038, #12082, #8068, #14574, #19726, #7881 ) ) ;
#18025=AXIS2_PLACEMENT_3D ( 'NONE', #11752, #826, #7073 ) ;
#18028=CARTESIAN_POINT ( 'NONE',  ( -31.34819206192207020, 65.74999999999998579, 2.481238266578628338 ) ) ;
#18032=CARTESIAN_POINT ( 'NONE',  ( 26.99999999999999645, 65.00000000000000000, -12.50000000000000000 ) ) ;
#18036=AXIS2_PLACEMENT_3D ( 'NONE', #15505, #15402, #14011 ) ;
#18046=EDGE_CURVE ( 'NONE', #1440, #1135, #7597, .T. ) ;
#18058=CARTESIAN_POINT ( 'NONE',  ( -15.99999999999999289, 79.99999999999998579, -12.50000000000000000 ) ) ;
#18062=EDGE_CURVE ( 'NONE', #8661, #5484, #1322, .T. ) ;
#18068=CARTESIAN_POINT ( 'NONE',  ( 30.00000000000000000, 0.000000000000000000, 28.99999999999999645 ) ) ;
#18078=CARTESIAN_POINT ( 'NONE',  ( -27.75418142457269255, 9.358687574860853786, -4.265973664729101777 ) ) ;
#18082=CARTESIAN_POINT ( 'NONE',  ( -10.76567231371678268, 45.28977633731097541, -11.35779591101546870 ) ) ;
#18084=EDGE_CURVE ( 'NONE', #4912, #3287, #13167, .T. ) ;
#18086=ORIENTED_EDGE ( 'NONE', *, *, #8425, .T. ) ;
#18088=CARTESIAN_POINT ( 'NONE',  ( 1.421481300724954044, 54.47125872025552695, -1.791815321364545799 ) ) ;
#18095=ORIENTED_EDGE ( 'NONE', *, *, #1283, .F. ) ;
#18101=ORIENTED_EDGE ( 'NONE', *, *, #9247, .T. ) ;
#18102=ORIENTED_EDGE ( 'NONE', *, *, #583, .T. ) ;
#18103=CARTESIAN_POINT ( 'NONE',  ( -19.99317890361201577, 61.82300078473741678, -3.011576861204080746 ) ) ;
#18105=CARTESIAN_POINT ( 'NONE',  ( -11.72929844504693442, 63.53565811406050301, -2.601344003386943715 ) ) ;
#18109=ADVANCED_FACE ( 'NONE', ( #9664 ), #15496, .F. ) ;
#18114=CARTESIAN_POINT ( 'NONE',  ( -33.02519701587559098, 51.39208029789107002, -6.179649924386284354 ) ) ;
#18129=CARTESIAN_POINT ( 'NONE',  ( -29.98061410047647257, 65.74999999999995737, 2.827122728375906835 ) ) ;
#18130=ORIENTED_EDGE ( 'NONE', *, *, #8178, .T. ) ;
#18135=ORIENTED_EDGE ( 'NONE', *, *, #9858, .F. ) ;
#18136=CARTESIAN_POINT ( 'NONE',  ( 30.00000000000000000, 5.000000000000000000, 30.00000000000000000 ) ) ;
#18146=ORIENTED_EDGE ( 'NONE', *, *, #16424, .T. ) ;
#18152=CIRCLE ( 'NONE', #9002, 9.999999999999998224 ) ;
#18153=ORIENTED_EDGE ( 'NONE', *, *, #13219, .T. ) ;
#18156=AXIS2_PLACEMENT_3D ( 'NONE', #17379, #11013, #2859 ) ;
#18159=CARTESIAN_POINT ( 'NONE',  ( -20.05080448500343238, 80.00000000000873968, -11.83620004860030939 ) ) ;
#18173=CARTESIAN_POINT ( 'NONE',  ( 0.03950703498306113587, 78.52235084885757033, -5.999488569659739312 ) ) ;
#18174=ORIENTED_EDGE ( 'NONE', *, *, #324, .F. ) ;
#18176=DIRECTION ( 'NONE',  ( 0.000000000000000000, 0.000000000000000000, -1.000000000000000000 ) ) ;
#18178=CARTESIAN_POINT ( 'NONE',  ( -33.23742054212824826, 77.39904134002362923, -4.045748805519247426 ) ) ;
#18180=CARTESIAN_POINT ( 'NONE',  ( -29.99999999999999645, 5.000000000000000000, 4.650073815093233698 ) ) ;
#18185=CARTESIAN_POINT ( 'NONE',  ( -9.743283712094267912, 45.17557351322050607, -10.82820226318459333 ) ) ;
#18189=CARTESIAN_POINT ( 'NONE',  ( 1.482111447062408827, 53.96832415390036886, -2.310166060002879274 ) ) ;
#18190=CARTESIAN_POINT ( 'NONE',  ( 1.494707070328831433, 76.40691198588817201, -2.756354051672949002 ) ) ;
#18193=CARTESIAN_POINT ( 'NONE',  ( -35.00000000000000000, 64.25000000000000000, 2.481238266578627449 ) ) ;
#18213=CARTESIAN_POINT ( 'NONE',  ( -33.48858877339391427, 53.74629247648528008, -2.576042629322002675 ) ) ;
#18215=ORIENTED_EDGE ( 'NONE', *, *, #702, .F. ) ;
#18233=AXIS2_PLACEMENT_3D ( 'NONE', #15903, #1274, #19656 ) ;
#18251=CARTESIAN_POINT ( 'NONE',  ( -12.45378882924321395, 69.43579287346189233, -3.531915534904312093 ) ) ;
#18269=FACE_OUTER_BOUND ( 'NONE', #12006, .T. ) ;
#18272=CARTESIAN_POINT ( 'NONE',  ( -13.41585758817372920, 79.99915570215716798, -12.30640999581525286 ) ) ;
#18280=CARTESIAN_POINT ( 'NONE',  ( -28.39160343344309112, 8.714752148389077746, 1.677005692623972699 ) ) ;
#18286=CARTESIAN_POINT ( 'NONE',  ( -3.536038244605083314, 48.22321216239767949, -1.121469025438518452 ) ) ;
#18290=CARTESIAN_POINT ( 'NONE',  ( -3.238679877191993128, 60.93978609069553443, 1.964649670197885278 ) ) ;
#18291=CARTESIAN_POINT ( 'NONE',  ( -6.040364182935697102, 79.85300711528874729, -10.39706325934435327 ) ) ;
#18301=CIRCLE ( 'NONE', #3068, 11.00000000000002665 ) ;
#18316=ORIENTED_EDGE ( 'NONE', *, *, #17705, .F. ) ;
#18322=CARTESIAN_POINT ( 'NONE',  ( -31.60861962881361720, 50.39374029569145108, -9.070721203488703921 ) ) ;
#18334=FACE_BOUND ( 'NONE', #4741, .T. ) ;
#18336=ADVANCED_FACE ( 'NONE', ( #14666, #6454 ), #12850, .T. ) ;
#18341=VECTOR ( 'NONE', #2175, 1000.000000000000000 ) ;
#18343=VECTOR ( 'NONE', #4279, 1000.000000000000000 ) ;
#18351=CARTESIAN_POINT ( 'NONE',  ( -28.93885174497882673, 72.78546382685756555, 0.3359787457726054472 ) ) ;
#18354=LINE ( 'NONE', #2242, #7842 ) ;
#18371=CARTESIAN_POINT ( 'NONE',  ( -21.54135399647558202, 79.97447990077583313, -11.55951008316331574 ) ) ;
#18381=VERTEX_POINT ( 'NONE', #17825 ) ;
#18385=CARTESIAN_POINT ( 'NONE',  ( -6.484348779698995813, 79.99999999992091659, -8.118105310438910038 ) ) ;
#18389=FACE_OUTER_BOUND ( 'NONE', #7223, .T. ) ;
#18393=CARTESIAN_POINT ( 'NONE',  ( -25.99999999999998934, 9.999999999999994671, 7.500000000000008882 ) ) ;
#18401=CARTESIAN_POINT ( 'NONE',  ( -0.1451441909484942616, 63.40414104109810722, 2.432067769318205119 ) ) ;
#18408=ORIENTED_EDGE ( 'NONE', *, *, #13170, .F. ) ;
#18412=ORIENTED_EDGE ( 'NONE', *, *, #15780, .F. ) ;
#18413=ADVANCED_FACE ( 'NONE', ( #17619 ), #9645, .F. ) ;
#18426=CARTESIAN_POINT ( 'NONE',  ( -30.38872702552290761, 50.11721826652506451, -10.60405991245520418 ) ) ;
#18438=ORIENTED_EDGE ( 'NONE', *, *, #19135, .F. ) ;
#18448=B_SPLINE_CURVE_WITH_KNOTS ( 'NONE', 3,
 ( #2808, #17112, #17009, #15846, #1212, #9140, #7663, #2601, #13833, #895, #19024, #18806, #10961, #9042, #6448, #4497, #1111, #15544, #1002, #10735 ),
 .UNSPECIFIED., .F., .F.,
 ( 4, 2, 2, 2, 2, 2, 2, 2, 2, 4 ),
 ( 0.000000000000000000, 0.0009877350076376205726, 0.001975470015275241145, 0.002963205022912861718, 0.003950940030550482290, 0.004938675038188102863, 0.005926410045825723436, 0.006420277549644531553, 0.006914145053463339671, 0.007901880061100961111 ),
 .UNSPECIFIED. ) ;
#18473=CARTESIAN_POINT ( 'NONE',  ( -23.80213736597611884, 79.89664383654029223, -10.58772689523770083 ) ) ;
#18481=CARTESIAN_POINT ( 'NONE',  ( -27.50180796992659182, 64.24999999999997158, 4.917728941844616841 ) ) ;
#18492=ORIENTED_EDGE ( 'NONE', *, *, #11932, .F. ) ;
#18496=EDGE_CURVE ( 'NONE', #8008, #12002, #2133, .T. ) ;
#18499=CARTESIAN_POINT ( 'NONE',  ( -28.48655238447041071, 8.589452128384102991, 0.6702984623187877578 ) ) ;
#18501=LINE ( 'NONE', #12037, #829 ) ;
#18504=AXIS2_PLACEMENT_3D ( 'NONE', #17953, #3418, #9766 ) ;
#18521=ORIENTED_EDGE ( 'NONE', *, *, #18722, .T. ) ;
#18530=ORIENTED_EDGE ( 'NONE', *, *, #6963, .T. ) ;
#18531=CARTESIAN_POINT ( 'NONE',  ( -15.99999999999999289, 5.000000000000000000, 0.000000000000000000 ) ) ;
#18533=FACE_OUTER_BOUND ( 'NONE', #6112, .T. ) ;
#18534=CARTESIAN_POINT ( 'NONE',  ( -15.53172565362767266, 50.47638478530413408, -16.25028014708374613 ) ) ;
#18537=CARTESIAN_POINT ( 'NONE',  ( -27.30844811143078132, 63.47441656769112228, 5.326305501724396763 ) ) ;
#18538=AXIS2_PLACEMENT_3D ( 'NONE', #409, #17796, #6857 ) ;
#18546=ORIENTED_EDGE ( 'NONE', *, *, #6429, .F. ) ;
#18556=VECTOR ( 'NONE', #12482, 1000.000000000000000 ) ;
#18557=DIRECTION ( 'NONE',  ( 0.000000000000000000, 1.000000000000000000, 0.000000000000000000 ) ) ;
#18562=CARTESIAN_POINT ( 'NONE',  ( 30.10683012259193703, 0.000000000000000000, 0.000000000000000000 ) ) ;
#18563=CARTESIAN_POINT ( 'NONE',  ( -27.98480658401470578, 74.73312780907578201, 3.553696893467978679 ) ) ;
#18594=CIRCLE ( 'NONE', #12167, 4.999999999999989342 ) ;
#18598=CARTESIAN_POINT ( 'NONE',  ( -33.39910372087116031, 76.99404724422815605, -3.489146652177067764 ) ) ;
#18608=CARTESIAN_POINT ( 'NONE',  ( -3.350687231550970147, 64.83636698465690529, 2.499114823701145571 ) ) ;
#18609=CIRCLE ( 'NONE', #1380, 12.50000000000000000 ) ;
#18611=DIRECTION ( 'NONE',  ( 0.000000000000000000, 0.000000000000000000, -1.000000000000000000 ) ) ;
#18622=ORIENTED_EDGE ( 'NONE', *, *, #20480, .F. ) ;
#18629=CARTESIAN_POINT ( 'NONE',  ( -19.90320481066766689, 68.50873499742380091, -3.129598480498279045 ) ) ;
#18630=VECTOR ( 'NONE', #7236, 1000.000000000000000 ) ;
#18634=ADVANCED_FACE ( 'NONE', ( #753 ), #15398, .T. ) ;
#18637=CARTESIAN_POINT ( 'NONE',  ( -22.59901147243187580, 50.26217980097501936, -15.30251921331534426 ) ) ;
#18639=DIRECTION ( 'NONE',  ( 0.000000000000000000, 0.000000000000000000, -1.000000000000000000 ) ) ;
#18640=CARTESIAN_POINT ( 'NONE',  ( -27.41141517789169768, 61.16284628816836744, 5.102783302178296232 ) ) ;
#18642=ORIENTED_EDGE ( 'NONE', *, *, #19437, .F. ) ;
#18645=AXIS2_PLACEMENT_3D ( 'NONE', #16153, #19417, #6468 ) ;
#18649=CARTESIAN_POINT ( 'NONE',  ( -23.72779897500315727, 50.18955727852706872, -14.96816017130344889 ) ) ;
#18656=CARTESIAN_POINT ( 'NONE',  ( -11.10102051443364779, 14.09941697557065332, 0.9999999999999991118 ) ) ;
#18678=CIRCLE ( 'NONE', #11913, 12.50000000000000000 ) ;
#18692=AXIS2_PLACEMENT_3D ( 'NONE', #12985, #16369, #14384 ) ;
#18693=CIRCLE ( 'NONE', #4794, 14.00000000000000178 ) ;
#18698=CARTESIAN_POINT ( 'NONE',  ( -20.89897948556633978, 16.09941697557071905, 0.9999999999999991118 ) ) ;
#18709=CARTESIAN_POINT ( 'NONE',  ( -15.99999999999999289, 80.00000000000000000, -12.50000000000000000 ) ) ;
#18717=ORIENTED_EDGE ( 'NONE', *, *, #14731, .T. ) ;
#18722=EDGE_CURVE ( 'NONE', #10584, #6984, #17935, .T. ) ;
#18723=LINE ( 'NONE', #3871, #19957 ) ;
#18724=CARTESIAN_POINT ( 'NONE',  ( 26.99999999999999645, 64.25000000000000000, -2.528164662410438357 ) ) ;
#18731=ORIENTED_EDGE ( 'NONE', *, *, #702, .T. ) ;
#18736=CARTESIAN_POINT ( 'NONE',  ( -16.35862578389054889, 71.60341624250784776, -4.990290896351837091 ) ) ;
#18743=CARTESIAN_POINT ( 'NONE',  ( -30.11049765362162134, 50.08318726096587170, -10.89667398352873029 ) ) ;
#18747=CARTESIAN_POINT ( 'NONE',  ( -35.00000000000000000, 65.74999999999997158, 2.481238266578629226 ) ) ;
#18753=DIRECTION ( 'NONE',  ( 0.000000000000000000, 0.000000000000000000, -1.000000000000000000 ) ) ;
#18759=CARTESIAN_POINT ( 'NONE',  ( 1.492765116366511435, 53.68125995765908698, -2.649088797068363199 ) ) ;
#18768=DIRECTION ( 'NONE',  ( 0.000000000000000000, -1.000000000000000000, 0.000000000000000000 ) ) ;
#18772=CARTESIAN_POINT ( 'NONE',  ( -27.55795892725420160, 70.83821676753269969, 4.766221741044114779 ) ) ;
#18775=CARTESIAN_POINT ( 'NONE',  ( -28.94270596280446739, 74.04855861174519305, -0.5148205403795984569 ) ) ;
#18778=ORIENTED_EDGE ( 'NONE', *, *, #13219, .F. ) ;
#18787=EDGE_LOOP ( 'NONE', ( #4536, #5515 ) ) ;
#18788=CYLINDRICAL_SURFACE ( 'NONE', #12807, 9.999999999999998224 ) ;
#18790=FACE_BOUND ( 'NONE', #18787, .T. ) ;
#18798=ORIENTED_EDGE ( 'NONE', *, *, #8425, .F. ) ;
#18806=CARTESIAN_POINT ( 'NONE',  ( -13.48852428594715747, 10.76355435230335011, 12.24827897062957227 ) ) ;
#18807=DIRECTION ( 'NONE',  ( 6.608470384673549052E-16, -1.000000000000000000, 0.000000000000000000 ) ) ;
#18810=DIRECTION ( 'NONE',  ( 0.000000000000000000, 1.000000000000000000, 0.000000000000000000 ) ) ;
#18811=AXIS2_PLACEMENT_3D ( 'NONE', #16873, #13701, #8812 ) ;
#18813=VECTOR ( 'NONE', #9000, 1000.000000000000000 ) ;
#18816=DIRECTION ( 'NONE',  ( 1.000000000000000000, 0.000000000000000000, 0.000000000000000000 ) ) ;
#18822=FACE_OUTER_BOUND ( 'NONE', #7683, .T. ) ;
#18823=CARTESIAN_POINT ( 'NONE',  ( -14.99999999999999645, -10.00000000000000000, -30.00000000000000000 ) ) ;
#18824=CYLINDRICAL_SURFACE ( 'NONE', #1708, 5.000000000000000000 ) ;
#18846=CARTESIAN_POINT ( 'NONE',  ( -18.93604315306787100, 49.50911328882459372, -12.15750417611710787 ) ) ;
#18855=CARTESIAN_POINT ( 'NONE',  ( -3.510843195177423492, 80.00000000000000000, 0.5205403966592451193 ) ) ;
#18863=CARTESIAN_POINT ( 'NONE',  ( -33.35732806943984485, 52.10193024710888210, -4.832466544100828543 ) ) ;
#18864=CARTESIAN_POINT ( 'NONE',  ( -26.77079800181776648, 9.903286195278038662, -6.378645726547156336 ) ) ;
#18871=CARTESIAN_POINT ( 'NONE',  ( -11.03378583276534108, 15.76606607271690841, 11.47134211267085391 ) ) ;
#18888=CARTESIAN_POINT ( 'NONE',  ( -4.574195094169405174, 69.03990363093106453, 5.071150534606958971 ) ) ;
#18900=ORIENTED_EDGE ( 'NONE', *, *, #7939, .F. ) ;
#18903=CARTESIAN_POINT ( 'NONE',  ( 27.00000000000002487, 65.74999999999997158, 2.481238266578629226 ) ) ;
#18911=CARTESIAN_POINT ( 'NONE',  ( -28.50080181521929745, 80.00000000000000000, 0.2411454413934158159 ) ) ;
#18912=ORIENTED_EDGE ( 'NONE', *, *, #19357, .T. ) ;
#18915=DIRECTION ( 'NONE',  ( -1.000000000000000000, 0.000000000000000000, 0.000000000000000000 ) ) ;
#18925=CARTESIAN_POINT ( 'NONE',  ( -11.10102051443364779, 16.09941697557071905, 0.9999999999999997780 ) ) ;
#18944=CARTESIAN_POINT ( 'NONE',  ( -25.65654271851453316, 45.04382983066486190, -7.944781169143150912 ) ) ;
#18955=CARTESIAN_POINT ( 'NONE',  ( 0.9782604970530670574, 77.74400922168841532, -4.586390192071695182 ) ) ;
#18961=CARTESIAN_POINT ( 'NONE',  ( -33.32166605174446516, 55.08543698672535527, -1.237103341644910648 ) ) ;
#18963=CARTESIAN_POINT ( 'NONE',  ( -26.41437051192821883, 9.999999999999996447, 6.947505984095691645 ) ) ;
#18968=EDGE_CURVE ( 'NONE', #12002, #4596, #18594, .T. ) ;
#18981=VECTOR ( 'NONE', #10297, 1000.000000000000000 ) ;
#18991=CARTESIAN_POINT ( 'NONE',  ( -3.056599057715243095, 73.00589460461357305, 0.1996236911402666236 ) ) ;
#19012=VECTOR ( 'NONE', #11268, 1000.000000000000000 ) ;
#19024=CARTESIAN_POINT ( 'NONE',  ( -12.94451012642581667, 11.12812038848359641, 12.12401870821426719 ) ) ;
#19025=CARTESIAN_POINT ( 'NONE',  ( -16.00000000000007105, 58.38562172233837089, -4.999999999999997335 ) ) ;
#19033=CARTESIAN_POINT ( 'NONE',  ( -31.82323003959540486, 65.74999999999997158, 2.481238266578629226 ) ) ;
#19039=CARTESIAN_POINT ( 'NONE',  ( -29.99999999999999645, 5.000000000000000000, 15.00000000000000000 ) ) ;
#19050=DIRECTION ( 'NONE',  ( -0.000000000000000000, 1.000000000000000000, -0.000000000000000000 ) ) ;
#19056=CARTESIAN_POINT ( 'NONE',  ( -15.99999999999999289, 20.09941697557067997, 12.50000000000000000 ) ) ;
#19057=CARTESIAN_POINT ( 'NONE',  ( -0.4109910671737397325, 50.38691911710247240, -9.099745271904268407 ) ) ;
#19067=CARTESIAN_POINT ( 'NONE',  ( -2.528458586775709893, 77.37584602520038857, -3.922623763562873123 ) ) ;
#19072=CARTESIAN_POINT ( 'NONE',  ( -12.10766532132493367, 50.39772591864724660, -15.93512085822366231 ) ) ;
#19075=VERTEX_POINT ( 'NONE', #825 ) ;
#19087=EDGE_CURVE ( 'NONE', #15321, #9010, #8970, .T. ) ;
#19096=CARTESIAN_POINT ( 'NONE',  ( -3.215901834620719768, 75.81673797945757087, -2.071606702244279674 ) ) ;
#19097=CARTESIAN_POINT ( 'NONE',  ( -14.99999999999999645, -10.00000000000000000, 15.00000000000000000 ) ) ;
#19108=CARTESIAN_POINT ( 'NONE',  ( 0.2950380200214504645, 60.04495121932129820, 1.663291502479429251 ) ) ;
#19110=DIRECTION ( 'NONE',  ( 0.000000000000000000, 0.000000000000000000, -1.000000000000000000 ) ) ;
#19118=EDGE_CURVE ( 'NONE', #17847, #11795, #1035, .T. ) ;
#19119=CARTESIAN_POINT ( 'NONE',  ( -15.99999999999999289, 80.00000000000000000, -4.999999999999993783 ) ) ;
#19121=CARTESIAN_POINT ( 'NONE',  ( -18.48100260771138537, 20.09941697557067641, 4.999999999999990230 ) ) ;
#19126=( LENGTH_UNIT ( ) NAMED_UNIT ( * ) SI_UNIT ( .MILLI., .METRE. ) );
#19127=CARTESIAN_POINT ( 'NONE',  ( -15.99999999999999289, 80.00000000000000000, 4.999999999999993783 ) ) ;
#19132=ORIENTED_EDGE ( 'NONE', *, *, #13893, .F. ) ;
#19135=EDGE_CURVE ( 'NONE', #13669, #7321, #14232, .T. ) ;
#19146=DIRECTION ( 'NONE',  ( 0.000000000000000000, -1.000000000000000000, 0.000000000000000000 ) ) ;
#19154=AXIS2_PLACEMENT_3D ( 'NONE', #19097, #4570, #11036 ) ;
#19156=CARTESIAN_POINT ( 'NONE',  ( -5.258301051201804910, 51.04712924960224285, -6.516085000401124816 ) ) ;
#19167=CARTESIAN_POINT ( 'NONE',  ( -3.376929201035539840, 76.35052269458216756, -2.692414605357460466 ) ) ;
#19173=CARTESIAN_POINT ( 'NONE',  ( -32.22615568004599851, 60.40488302444183688, 1.799529103756865478 ) ) ;
#19175=DIRECTION ( 'NONE',  ( 0.000000000000000000, 0.000000000000000000, 1.000000000000000000 ) ) ;
#19179=CARTESIAN_POINT ( 'NONE',  ( -0.03591081202477939410, 67.75983095507352516, 2.252573492070593986 ) ) ;
#19184=CARTESIAN_POINT ( 'NONE',  ( -27.39676811513723109, 61.45283151330974647, 5.134886483425054493 ) ) ;
#19188=DIRECTION ( 'NONE',  ( 0.000000000000000000, 0.000000000000000000, 1.000000000000000000 ) ) ;
#19194=EDGE_CURVE ( 'NONE', #8955, #8547, #9106, .T. ) ;
#19216=ORIENTED_EDGE ( 'NONE', *, *, #15660, .T. ) ;
#19221=LINE ( 'NONE', #7868, #10814 ) ;
#19234=CARTESIAN_POINT ( 'NONE',  ( -28.16330156462496603, 79.99999999984028420, -2.903060217166834267 ) ) ;
#19248=CIRCLE ( 'NONE', #10080, 9.999999999999998224 ) ;
#19255=ORIENTED_EDGE ( 'NONE', *, *, #17292, .F. ) ;
#19261=CARTESIAN_POINT ( 'NONE',  ( -5.379344836516867900, 50.95069562376034611, -6.689558405576774724 ) ) ;
#19265=LINE ( 'NONE', #14405, #2245 ) ;
#19269=DIRECTION ( 'NONE',  ( 1.000000000000000000, 0.000000000000000000, 0.000000000000000000 ) ) ;
#19271=CARTESIAN_POINT ( 'NONE',  ( -11.94919551499654808, 80.00000000000871125, -11.83620004860075703 ) ) ;
#19277=CARTESIAN_POINT ( 'NONE',  ( -33.09260109148557660, 56.28423912749347835, -0.2677176956847754363 ) ) ;
#19287=LINE ( 'NONE', #9625, #6858 ) ;
#19289=CARTESIAN_POINT ( 'NONE',  ( -28.72625095155510522, 68.32062926339966680, 2.141136792363286911 ) ) ;
#19290=DIRECTION ( 'NONE',  ( 0.000000000000000000, 0.000000000000000000, -1.000000000000000000 ) ) ;
#19324=( NAMED_UNIT ( * ) SI_UNIT ( $, .STERADIAN. ) SOLID_ANGLE_UNIT ( ) );
#19330=CARTESIAN_POINT ( 'NONE',  ( -32.28295608689890628, 78.37037279069637918, -5.691146419800033662 ) ) ;
#19348=DIRECTION ( 'NONE',  ( 0.7071067811865432429, 0.000000000000000000, -0.7071067811865517916 ) ) ;
#19351=AXIS2_PLACEMENT_3D ( 'NONE', #3815, #2135, #16860 ) ;
#19353=DIRECTION ( 'NONE',  ( 0.000000000000000000, 1.000000000000000000, 0.000000000000000000 ) ) ;
#19355=ORIENTED_EDGE ( 'NONE', *, *, #618, .T. ) ;
#19356=CARTESIAN_POINT ( 'NONE',  ( -34.00000000000000711, 65.00000000000000000, -12.50000000000000000 ) ) ;
#19357=EDGE_CURVE ( 'NONE', #5157, #15623, #3461, .T. ) ;
#19359=CARTESIAN_POINT ( 'NONE',  ( -4.864993619586824636, 45.51589215631262419, -5.690233592220027781 ) ) ;
#19364=VECTOR ( 'NONE', #10881, 1000.000000000000000 ) ;
#19371=CARTESIAN_POINT ( 'NONE',  ( -12.38627653609458257, 79.99792423946917097, -12.24236967450151958 ) ) ;
#19375=DIRECTION ( 'NONE',  ( 1.000000000000000000, -0.000000000000000000, 0.000000000000000000 ) ) ;
#19381=ORIENTED_EDGE ( 'NONE', *, *, #6930, .F. ) ;
#19390=CARTESIAN_POINT ( 'NONE',  ( 44.00000000000000000, 0.000000000000000000, -15.00000000000000355 ) ) ;
#19396=ORIENTED_EDGE ( 'NONE', *, *, #13033, .T. ) ;
#19399=ADVANCED_FACE ( 'NONE', ( #20088 ), #17798, .F. ) ;
#19402=EDGE_CURVE ( 'NONE', #8219, #4596, #10943, .T. ) ;
#19417=DIRECTION ( 'NONE',  ( 0.000000000000000000, -1.000000000000000000, 0.000000000000000000 ) ) ;
#19426=CARTESIAN_POINT ( 'NONE',  ( -33.07802712247563193, 73.66227117401376745, -0.2439945722892326863 ) ) ;
#19437=EDGE_CURVE ( 'NONE', #11977, #11320, #2891, .T. ) ;
#19438=ORIENTED_EDGE ( 'NONE', *, *, #15677, .T. ) ;
#19442=CARTESIAN_POINT ( 'NONE',  ( -33.48481952675158624, 80.00000000000001421, 0.7287565553229297111 ) ) ;
#19443=CARTESIAN_POINT ( 'NONE',  ( -29.99999999999996447, 5.000000000000006217, -9.730120459829299406 ) ) ;
#19447=B_SPLINE_CURVE_WITH_KNOTS ( 'NONE', 3,
 ( #7397, #12819, #94, #18103, #1783, #16107, #12922, #8225, #6525, #3159, #6629, #4947, #5152, #9914, #3569, #13123, #11639, #10015, #8333, #1884, #16508, #17692 ),
 .UNSPECIFIED., .F., .F.,
 ( 4, 2, 2, 2, 2, 2, 2, 2, 2, 2, 4 ),
 ( 0.000000000000000000, 0.002138836336596521351, 0.003208254504894782026, 0.004277672673193042702, 0.004812381757342181279, 0.005347090841491319857, 0.006416509009789597880, 0.006951218093938736457, 0.007485927178087873300, 0.008020636262237011010, 0.008555345346386149588 ),
 .UNSPECIFIED. ) ;
#19450=CARTESIAN_POINT ( 'NONE',  ( -11.12092984962295539, 45.32949789690962206, -11.51493324710881971 ) ) ;
#19451=CARTESIAN_POINT ( 'NONE',  ( -6.842857967119176266, 50.10839126059149606, -14.33286777257530709 ) ) ;
#19452=CARTESIAN_POINT ( 'NONE',  ( 0.6607651890765847691, 78.07072705852067429, -5.138138717405499101 ) ) ;
#19455=CONICAL_SURFACE ( 'NONE', #12428, 14.99999999999999645, 0.7853981633974543852 ) ;
#19456=ORIENTED_EDGE ( 'NONE', *, *, #9899, .F. ) ;
#19460=DIRECTION ( 'NONE',  ( 0.000000000000000000, 0.000000000000000000, -1.000000000000000000 ) ) ;
#19469=FACE_OUTER_BOUND ( 'NONE', #2009, .T. ) ;
#19470=AXIS2_PLACEMENT_3D ( 'NONE', #5463, #8440, #720 ) ;
#19477=CARTESIAN_POINT ( 'NONE',  ( -28.66803663422406601, 63.25105461977041443, 2.419216852106436999 ) ) ;
#19478=CARTESIAN_POINT ( 'NONE',  ( -20.83667610223213629, 16.40927555158100759, 11.52655978026935024 ) ) ;
#19482=CARTESIAN_POINT ( 'NONE',  ( 27.66668267600675435, 65.75000000000001421, 1.813692929321165437 ) ) ;
#19484=ORIENTED_EDGE ( 'NONE', *, *, #675, .T. ) ;
#19486=ORIENTED_EDGE ( 'NONE', *, *, #19402, .T. ) ;
#19494=CARTESIAN_POINT ( 'NONE',  ( -14.99999999999999645, 5.000000000000000000, -15.00000000000000000 ) ) ;
#19499=VECTOR ( 'NONE', #9352, 1000.000000000000000 ) ;
#19500=DIRECTION ( 'NONE',  ( 0.000000000000000000, -0.000000000000000000, -1.000000000000000000 ) ) ;
#19512=CARTESIAN_POINT ( 'NONE',  ( -15.99999999999999289, 80.00000000000000000, 0.000000000000000000 ) ) ;
#19514=CARTESIAN_POINT ( 'NONE',  ( -11.71793669819365569, 66.46870624085923396, -2.582219875156729127 ) ) ;
#19528=CARTESIAN_POINT ( 'NONE',  ( -31.50431546803533678, 78.79719334215234028, -6.605250029488051844 ) ) ;
#19535=B_SPLINE_CURVE_WITH_KNOTS ( 'NONE', 3,
 ( #7245, #8733, #13628, #15127, #18598, #18178, #4068, #14910, #5325, #20080, #6826, #13411, #19859, #11715, #16035, #9536, #20872, #1601, #20284, #1005, #15, #9044, #1396, #7345, #13944, #9428, #13835, #6450, #12735, #5746, #12639, #18709 ),
 .UNSPECIFIED., .F., .F.,
 ( 4, 2, 2, 2, 2, 2, 2, 2, 2, 2, 2, 2, 2, 2, 2, 4 ),
 ( 0.000000000000000000, 0.0007065482847658889143, 0.001413096569531777829, 0.002826193139063555657, 0.003532741423829438825, 0.004239289708595322427, 0.005652386278127087896, 0.007065482847658845558, 0.008478579417190603221, 0.01130477255625412202, 0.01271786912578587794, 0.01413096569531763214, 0.01695715883438114399, 0.01978335197344465238, 0.02119644854297641004, 0.02260954511250816423 ),
 .UNSPECIFIED. ) ;
#19536=CARTESIAN_POINT ( 'NONE',  ( -15.99999999999999289, 80.00000000000000000, 0.000000000000000000 ) ) ;
#19543=DIRECTION ( 'NONE',  ( -0.000000000000000000, -1.000000000000000000, -0.000000000000000000 ) ) ;
#19553=CARTESIAN_POINT ( 'NONE',  ( -12.20066445503069019, 45.44343745760707520, -11.93361228997413725 ) ) ;
#19556=CARTESIAN_POINT ( 'NONE',  ( 1.121154864378749672, 56.12821655472171756, -0.3994926274425245061 ) ) ;
#19582=CARTESIAN_POINT ( 'NONE',  ( -28.93726274132100329, 55.68764042281951276, -0.7073738265182815121 ) ) ;
#19593=CARTESIAN_POINT ( 'NONE',  ( -0.1461903257121275057, 66.50634452888081682, 2.432944671161595185 ) ) ;
#19596=CARTESIAN_POINT ( 'NONE',  ( -33.99999999999997868, 65.00000000000000000, -22.50000000000000000 ) ) ;
#19603=VECTOR ( 'NONE', #17047, 1000.000000000000000 ) ;
#19608=DIRECTION ( 'NONE',  ( -0.000000000000000000, -1.000000000000000000, -0.000000000000000000 ) ) ;
#19635=DIRECTION ( 'NONE',  ( -0.000000000000000000, 1.000000000000000000, -0.000000000000000000 ) ) ;
#19639=CARTESIAN_POINT ( 'NONE',  ( -29.99999999999999645, 10.00000000000000000, 10.50000000000000000 ) ) ;
#19642=DIRECTION ( 'NONE',  ( 0.000000000000000000, -1.000000000000000000, 0.000000000000000000 ) ) ;
#19644=CONICAL_SURFACE ( 'NONE', #17968, 4.999999999999995559, 1.029744258676653867 ) ;
#19647=CARTESIAN_POINT ( 'NONE',  ( 30.00000000000000000, -10.00000000000000000, 30.00000000000000000 ) ) ;
#19653=CARTESIAN_POINT ( 'NONE',  ( -27.37662084148517039, 9.618015882392517923, -5.189762514993161879 ) ) ;
#19656=DIRECTION ( 'NONE',  ( 1.000000000000000000, 0.000000000000000000, 0.000000000000000000 ) ) ;
#19664=CARTESIAN_POINT ( 'NONE',  ( 1.274666701857165352, 51.86400000113221154, -5.249213278443415120 ) ) ;
#19665=CARTESIAN_POINT ( 'NONE',  ( -8.643231066280758768, 79.96312735385207304, -11.40287558748652863 ) ) ;
#19674=VECTOR ( 'NONE', #12710, 1000.000000000000000 ) ;
#19676=ORIENTED_EDGE ( 'NONE', *, *, #464, .F. ) ;
#19680=CARTESIAN_POINT ( 'NONE',  ( -13.43323294362767051, 59.26984403206416374, -4.299749073728320603 ) ) ;
#19691=CARTESIAN_POINT ( 'NONE',  ( -28.09246286469363341, 54.35809415438139069, 3.171690999751710205 ) ) ;
#19698=ORIENTED_EDGE ( 'NONE', *, *, #11877, .T. ) ;
#19699=CARTESIAN_POINT ( 'NONE',  ( -4.675850232754709346, 67.00845937185172829, 5.293280639217825545 ) ) ;
#19707=CARTESIAN_POINT ( 'NONE',  ( -29.54966092877796413, 65.74999999999997158, 3.021668726329258980 ) ) ;
#19719=LINE ( 'NONE', #4789, #19012 ) ;
#19726=ORIENTED_EDGE ( 'NONE', *, *, #15377, .F. ) ;
#19727=PRODUCT_DEFINITION ( 'UNKNOWN', '', #20938, #6176 ) ;
#19736=CARTESIAN_POINT ( 'NONE',  ( -20.12129706306810917, 79.99650906190643695, -12.16257741986414231 ) ) ;
#19741=CARTESIAN_POINT ( 'NONE',  ( 30.00000000000000355, -10.00000000000000000, -15.00000000000000000 ) ) ;
#19746=AXIS2_PLACEMENT_3D ( 'NONE', #17094, #10496, #2356 ) ;
#19749=DIRECTION ( 'NONE',  ( 0.000000000000000000, 0.000000000000000000, -1.000000000000000000 ) ) ;
#19753=CARTESIAN_POINT ( 'NONE',  ( 0.2829560868989292599, 78.37037279069626550, -5.691146419799841816 ) ) ;
#19755=ORIENTED_EDGE ( 'NONE', *, *, #7680, .F. ) ;
#19762=CARTESIAN_POINT ( 'NONE',  ( -29.99999999999999645, 5.000000000000000888, -10.11947335595186281 ) ) ;
#19767=CARTESIAN_POINT ( 'NONE',  ( -12.93758089954634372, 45.51191724327595978, -12.14335867266129299 ) ) ;
#19769=CARTESIAN_POINT ( 'NONE',  ( 28.00000000000001066, 64.25000000000000000, 1.479896280015810639 ) ) ;
#19770=CARTESIAN_POINT ( 'NONE',  ( 0.7229626692810823263, 57.94382164277974567, 0.7560164722777046320 ) ) ;
#19771=CARTESIAN_POINT ( 'NONE',  ( 1.076391949077661669, 77.63996874865388520, -4.412329984541580430 ) ) ;
#19772=ADVANCED_FACE ( 'NONE', ( #10056 ), #6946, .F. ) ;
#19780=CARTESIAN_POINT ( 'NONE',  ( -20.89897948556633978, 14.09941697557065332, 0.9999999999999991118 ) ) ;
#19782=ORIENTED_EDGE ( 'NONE', *, *, #3481, .F. ) ;
#19786=DIRECTION ( 'NONE',  ( 0.000000000000000000, 0.000000000000000000, -1.000000000000000000 ) ) ;
#19788=EDGE_CURVE ( 'NONE', #6578, #10554, #15087, .T. ) ;
#19789=DIRECTION ( 'NONE',  ( 0.000000000000000000, -0.000000000000000000, -1.000000000000000000 ) ) ;
#19793=VECTOR ( 'NONE', #501, 1000.000000000000000 ) ;
#19795=CARTESIAN_POINT ( 'NONE',  ( -28.22952087382082809, 47.05996708829931663, -2.604621190020335764 ) ) ;
#19813=DIRECTION ( 'NONE',  ( -0.000000000000000000, 1.000000000000000000, -0.000000000000000000 ) ) ;
#19849=DIRECTION ( 'NONE',  ( 0.000000000000000000, 1.000000000000000000, 0.000000000000000000 ) ) ;
#19853=CARTESIAN_POINT ( 'NONE',  ( -9.066344050852512382, 79.93797039651413172, -11.02074839553305985 ) ) ;
#19857=CARTESIAN_POINT ( 'NONE',  ( 44.00000000000000000, -10.00000000000000000, -15.00000000000000355 ) ) ;
#19859=CARTESIAN_POINT ( 'NONE',  ( -31.59797023739843880, 78.75485493504352519, -6.506575737150531502 ) ) ;
#19861=CARTESIAN_POINT ( 'NONE',  ( -28.50006506553908281, 8.570624926478151551, 0.3342343741539107738 ) ) ;
#19867=CARTESIAN_POINT ( 'NONE',  ( -3.692367643534749888, 52.45729905868842025, 2.215249628048927111 ) ) ;
#19868=VECTOR ( 'NONE', #19635, 1000.000000000000000 ) ;
#19871=CARTESIAN_POINT ( 'NONE',  ( -4.388108127469900310, 58.67718948633005027, 4.628796252570745118 ) ) ;
#19872=CARTESIAN_POINT ( 'NONE',  ( -7.329809494601250641, 79.91878874140672906, -10.93332899582966711 ) ) ;
#19888=DIRECTION ( 'NONE',  ( 0.000000000000000000, -1.000000000000000000, 0.000000000000000000 ) ) ;
#19893=CARTESIAN_POINT ( 'NONE',  ( -19.67966358621957923, 69.13720662105420445, -3.389612121674969725 ) ) ;
#19900=CARTESIAN_POINT ( 'NONE',  ( -31.81916350473495925, 50.47282605692874569, -8.748658904665091995 ) ) ;
#19907=VERTEX_POINT ( 'NONE', #7625 ) ;
#19910=ORIENTED_EDGE ( 'NONE', *, *, #11000, .F. ) ;
#19926=EDGE_LOOP ( 'NONE', ( #18622, #11269, #4637, #14517, #664 ) ) ;
#19927=CARTESIAN_POINT ( 'NONE',  ( -32.97264659046876289, 73.17878816827422384, 0.08443632837269006430 ) ) ;
#19933=CARTESIAN_POINT ( 'NONE',  ( -2.810302697974978781, 79.49366880382952161, -8.593311550919597863 ) ) ;
#19939=B_SPLINE_CURVE_WITH_KNOTS ( 'NONE', 3,
 ( #126, #6560, #12743, #20683, #6156, #12648, #19108, #11045, #4336, #12303, #2858, #1165, #8986, #17378, #5806, #18759, #14214, #17066, #15895, #7715, #11012, #4232, #2543, #15489, #4127, #14318, #20441, #10581, #9293, #948, #10679, #4440, #1367, #20334, #4544, #17165, #20753, #2752, #20641, #6221, #17481, #19072, #7391, #2958, #2647, #12611, #10787, #7818, #9399, #10900, #18649, #9090, #17267, #9193, #15699, #13882, #15797, #1266, #15589, #1056, #7505, #13997, #5905, #7613, #12405, #18863, #20540, #14103, #12501, #6115, #6011, #18961, #1785, #19277, #7919, #16008, #1677, #9714, #6322, #19173, #4648, #1574, #20847, #14418, #6527, #3161 ),
 .UNSPECIFIED., .F., .F.,
 ( 4, 2, 2, 2, 2, 2, 2, 2, 2, 2, 2, 2, 2, 2, 2, 2, 2, 2, 2, 2, 2, 2, 2, 2, 2, 2, 2, 2, 2, 2, 2, 2, 2, 2, 2, 2, 2, 2, 2, 2, 2, 2, 4 ),
 ( 0.000000000000000000, 0.002349933223531118325, 0.003524899835296677053, 0.004699866447062234914, 0.007049799670593371453, 0.008224766282358929315, 0.009399732894124488911, 0.01174966611765559076, 0.01292463272942114168, 0.01409959934118669087, 0.01527456595295224179, 0.01644953256471779271, 0.01879946578824888415, 0.01997443240001442813, 0.02114939901177997558, 0.02349933223531107049, 0.02467429884707661794, 0.02584926545884216192, 0.02819919868237325336, 0.03054913190590434480, 0.03289906512943543970, 0.03524899835296653461, 0.03759893157649762258, 0.03994886480002871054, 0.04229879802355979157, 0.04699866447062195363, 0.04934859769415304159, 0.05169853091768412956, 0.05404846414121521059, 0.05522343075298075110, 0.05639839736474629162, 0.05874833058827737264, 0.05992329720004292010, 0.06109826381180846061, 0.06344819703533953470, 0.06462316364710508909, 0.06579813025887064348, 0.06814806348240172451, 0.06932303009416727890, 0.07049799670593281942, 0.07284792992946390044, 0.07402289654122945484, 0.07519786315299499535 ),
 .UNSPECIFIED. ) ;
#19940=CARTESIAN_POINT ( 'NONE',  ( -15.99999999999999289, -9.999999999999994671, 0.000000000000000000 ) ) ;
#19941=VECTOR ( 'NONE', #20317, 1000.000000000000000 ) ;
#19944=CARTESIAN_POINT ( 'NONE',  ( -18.57603018928663019, 80.00000000000416378, -12.24234612424543478 ) ) ;
#19950=DIRECTION ( 'NONE',  ( 0.000000000000000000, 0.000000000000000000, -1.000000000000000000 ) ) ;
#19951=EDGE_CURVE ( 'NONE', #4749, #13189, #19981, .T. ) ;
#19955=LINE ( 'NONE', #12124, #18981 ) ;
#19957=VECTOR ( 'NONE', #20093, 1000.000000000000000 ) ;
#19958=CARTESIAN_POINT ( 'NONE',  ( -10.45864600352303420, 79.97447990077584734, -11.55951008316059614 ) ) ;
#19966=CARTESIAN_POINT ( 'NONE',  ( -26.09897484109792742, 5.223491560547939727, 7.368033551913470092 ) ) ;
#19979=CARTESIAN_POINT ( 'NONE',  ( -3.068708237237466108, 55.70095837538499950, -0.7135719611316724276 ) ) ;
#19981=B_SPLINE_CURVE_WITH_KNOTS ( 'NONE', 3,
 ( #13895, #12516, #2869, #854, #7304, #4140, #1281, #20241, #18772, #9415, #12830, #12721, #14747, #11024 ),
 .UNSPECIFIED., .F., .F.,
 ( 4, 2, 2, 2, 2, 2, 4 ),
 ( 1.510469127625910055E-17, 0.003820875137362821691, 0.005731312706044241860, 0.007641750274725663331, 0.01146262541208846811, 0.01337306298076985228, 0.01528350054945123472 ),
 .UNSPECIFIED. ) ;
#20002=CARTESIAN_POINT ( 'NONE',  ( 30.00000000000000000, -10.00000000000000000, 28.99999999999999645 ) ) ;
#20003=CARTESIAN_POINT ( 'NONE',  ( -18.56676705637232061, 70.73015596793582915, -4.299749073728317050 ) ) ;
#20009=FACE_OUTER_BOUND ( 'NONE', #228, .T. ) ;
#20010=CARTESIAN_POINT ( 'NONE',  ( -32.86183952535874653, 57.32352061648923325, 0.3918776291228620035 ) ) ;
#20014=VERTEX_POINT ( 'NONE', #6434 ) ;
#20016=CARTESIAN_POINT ( 'NONE',  ( 27.00000000000002487, 65.00000000000000000, -12.50000000000000000 ) ) ;
#20024=ADVANCED_FACE ( 'NONE', ( #12936 ), #9078, .F. ) ;
#20035=FACE_OUTER_BOUND ( 'NONE', #8815, .T. ) ;
#20037=DIRECTION ( 'NONE',  ( 1.000000000000000000, 0.000000000000000000, 0.000000000000000000 ) ) ;
#20043=PLANE ( 'NONE',  #13687 ) ;
#20055=ADVANCED_FACE ( 'NONE', ( #18822 ), #10641, .T. ) ;
#20070=VERTEX_POINT ( 'NONE', #20402 ) ;
#20073=CARTESIAN_POINT ( 'NONE',  ( -15.99999999999999289, 79.99999999999998579, -12.50000000000000000 ) ) ;
#20076=ORIENTED_EDGE ( 'NONE', *, *, #16615, .F. ) ;
#20078=DIRECTION ( 'NONE',  ( 0.000000000000000000, 1.000000000000000000, 0.000000000000000000 ) ) ;
#20080=CARTESIAN_POINT ( 'NONE',  ( -32.42127702560121350, 78.26431280098985610, -5.492938746012961282 ) ) ;
#20083=CARTESIAN_POINT ( 'NONE',  ( -26.92417954832534122, 9.835141389658375033, 6.084915548678262454 ) ) ;
#20088=FACE_OUTER_BOUND ( 'NONE', #12625, .T. ) ;
#20090=VERTEX_POINT ( 'NONE', #20498 ) ;
#20093=DIRECTION ( 'NONE',  ( 0.000000000000000000, 0.000000000000000000, -1.000000000000000000 ) ) ;
#20110=PLANE ( 'NONE',  #6596 ) ;
#20116=CARTESIAN_POINT ( 'NONE',  ( -24.74740475360116321, 50.13270831063489652, -14.49843712002114238 ) ) ;
#20118=DIRECTION ( 'NONE',  ( -1.000000000000000000, 0.000000000000000000, 0.000000000000000000 ) ) ;
#20119=CARTESIAN_POINT ( 'NONE',  ( -27.82037292730693778, 56.67161465046595481, 4.072047940184197579 ) ) ;
#20123=ORIENTED_EDGE ( 'NONE', *, *, #18046, .F. ) ;
#20128=EDGE_CURVE ( 'NONE', #9755, #9039, #14505, .T. ) ;
#20136=CYLINDRICAL_SURFACE ( 'NONE', #801, 9.999999999999998224 ) ;
#20137=CARTESIAN_POINT ( 'NONE',  ( -15.99999999999999289, 20.09941697557067997, 12.50000000000000000 ) ) ;
#20143=CARTESIAN_POINT ( 'NONE',  ( -33.06477925144887564, 73.59974835485031974, -0.1995438761935474647 ) ) ;
#20146=ORIENTED_EDGE ( 'NONE', *, *, #4972, .T. ) ;
#20147=CARTESIAN_POINT ( 'NONE',  ( -3.241054845510801918, 65.75000000000000000, 3.522626389267836444 ) ) ;
#20151=CARTESIAN_POINT ( 'NONE',  ( -11.00000000000000355, 15.09941697557068530, 15.00000000000000000 ) ) ;
#20174=CARTESIAN_POINT ( 'NONE',  ( -15.73951528932505894, 79.99999999999998579, -12.50000000001717204 ) ) ;
#20180=VECTOR ( 'NONE', #5796, 1000.000000000000000 ) ;
#20183=ADVANCED_FACE ( 'NONE', ( #17757 ), #7883, .F. ) ;
#20185=CARTESIAN_POINT ( 'NONE',  ( -30.00000000000032330, 4.999999999999686473, 1.877804259809431997 ) ) ;
#20190=AXIS2_PLACEMENT_3D ( 'NONE', #2607, #18810, #17219 ) ;
#20203=ORIENTED_EDGE ( 'NONE', *, *, #10117, .F. ) ;
#20212=CYLINDRICAL_SURFACE ( 'NONE', #18025, 4.999999999999990230 ) ;
#20213=CARTESIAN_POINT ( 'NONE',  ( -13.59909031749119102, 50.44595023350106544, -16.13088894857765965 ) ) ;
#20220=ORIENTED_EDGE ( 'NONE', *, *, #82, .T. ) ;
#20225=ORIENTED_EDGE ( 'NONE', *, *, #8634, .T. ) ;
#20232=B_SPLINE_CURVE_WITH_KNOTS ( 'NONE', 3,
 ( #2484, #10952, #14152, #2899, #993, #12449, #15428, #7758, #4171, #14042, #14261, #5849, #15537, #7437 ),
 .UNSPECIFIED., .F., .F.,
 ( 4, 2, 2, 2, 2, 2, 4 ),
 ( 0.000000000000000000, 0.001925163319758125494, 0.003850326639516250989, 0.007700653279032461211, 0.009625816598790543771, 0.01155097991854863067, 0.01540130655806476456 ),
 .UNSPECIFIED. ) ;
#20241=CARTESIAN_POINT ( 'NONE',  ( -27.68173125899994602, 72.07281518094384865, 4.467622400254045445 ) ) ;
#20243=EDGE_CURVE ( 'NONE', #15175, #6192, #1639, .T. ) ;
#20245=CARTESIAN_POINT ( 'NONE',  ( -32.82806271630868622, 72.52289824211611347, 0.4796438872512392426 ) ) ;
#20250=CARTESIAN_POINT ( 'NONE',  ( -0.6518013096703926257, 65.74999999999997158, 2.481238266578629226 ) ) ;
#20260=DIRECTION ( 'NONE',  ( 1.000000000000000000, 0.000000000000000000, 0.000000000000000000 ) ) ;
#20265=AXIS2_PLACEMENT_3D ( 'NONE', #19, #4979, #19500 ) ;
#20269=CARTESIAN_POINT ( 'NONE',  ( -28.23156009437249025, 64.24999999999998579, 3.993547312438774366 ) ) ;
#20272=CARTESIAN_POINT ( 'NONE',  ( -29.99999999999999645, 5.000000000000000000, 15.00000000000000000 ) ) ;
#20273=CARTESIAN_POINT ( 'NONE',  ( 30.10683012259193703, 5.000000000000000000, 4.999999999999997335 ) ) ;
#20284=CARTESIAN_POINT ( 'NONE',  ( -27.63293763622268528, 79.71668407523966948, -9.567129279037617451 ) ) ;
#20302=ORIENTED_EDGE ( 'NONE', *, *, #15677, .F. ) ;
#20312=CYLINDRICAL_SURFACE ( 'NONE', #4955, 4.999999999999989342 ) ;
#20317=DIRECTION ( 'NONE',  ( -0.000000000000000000, -1.000000000000000000, -0.000000000000000000 ) ) ;
#20320=CARTESIAN_POINT ( 'NONE',  ( -23.12579181598519540, 45.08735423564900913, -10.27585172372141287 ) ) ;
#20324=CARTESIAN_POINT ( 'NONE',  ( -28.34202942068278475, 47.50017047936148629, -2.003691985157042055 ) ) ;
#20330=FACE_OUTER_BOUND ( 'NONE', #5685, .T. ) ;
#20334=CARTESIAN_POINT ( 'NONE',  ( -4.143013757418743559, 50.00090654753341823, -12.78394331335679013 ) ) ;
#20340=DIRECTION ( 'NONE',  ( -0.000000000000000000, -1.000000000000000000, -0.000000000000000000 ) ) ;
#20343=EDGE_CURVE ( 'NONE', #2398, #3348, #15012, .T. ) ;
#20350=DIRECTION ( 'NONE',  ( 0.000000000000000000, 0.000000000000000000, -1.000000000000000000 ) ) ;
#20358=ORIENTED_EDGE ( 'NONE', *, *, #19194, .F. ) ;
#20368=CARTESIAN_POINT ( 'NONE',  ( -46.99999999999998579, 65.00000000000000000, -12.50000000000000000 ) ) ;
#20371=DIRECTION ( 'NONE',  ( 0.000000000000000000, 0.000000000000000000, -1.000000000000000000 ) ) ;
#20383=CARTESIAN_POINT ( 'NONE',  ( -14.95830009086074597, 79.99999999999985789, -12.45923801546573095 ) ) ;
#20388=CARTESIAN_POINT ( 'NONE',  ( 27.00000000000002487, 65.00000000000000000, -12.50000000000000000 ) ) ;
#20395=CARTESIAN_POINT ( 'NONE',  ( -34.66662763442661799, 64.25000000000000000, -1.859747928060479172 ) ) ;
#20396=CARTESIAN_POINT ( 'NONE',  ( -28.99999999999999289, -10.00000000000000000, -15.00000000000000000 ) ) ;
#20402=CARTESIAN_POINT ( 'NONE',  ( -14.99999999999999645, -10.00000000000000000, 30.00000000000000000 ) ) ;
#20422=CARTESIAN_POINT ( 'NONE',  ( -15.99999999999999289, 80.00000000000000000, 12.50000000000000000 ) ) ;
#20426=CARTESIAN_POINT ( 'NONE',  ( -25.48018294944744611, 50.26343215275641541, -8.155225720970078029 ) ) ;
#20441=CARTESIAN_POINT ( 'NONE',  ( -0.3030695078776163842, 50.42519578546549042, -8.938776343028093763 ) ) ;
#20442=CARTESIAN_POINT ( 'NONE',  ( -35.00000000000000000, 65.74999999999997158, -1.525597966176003961 ) ) ;
#20445=CARTESIAN_POINT ( 'NONE',  ( 1.442378013833077732, 75.57646748667872316, -1.814718499151617870 ) ) ;
#20450=CARTESIAN_POINT ( 'NONE',  ( -11.25987086420109229, 16.72409293340036385, 11.56718819196806791 ) ) ;
#20456=CARTESIAN_POINT ( 'NONE',  ( -32.20403829709411525, 69.52210068921769448, 1.838693167884530633 ) ) ;
#20458=CARTESIAN_POINT ( 'NONE',  ( -13.51899739228861463, 10.09941697557069595, 4.999999999999990230 ) ) ;
#20463=CARTESIAN_POINT ( 'NONE',  ( 0.8280627163074613106, 72.52289824211320024, 0.4796438872529771302 ) ) ;
#20480=EDGE_CURVE ( 'NONE', #18381, #9665, #15429, .T. ) ;
#20486=ORIENTED_EDGE ( 'NONE', *, *, #13273, .T. ) ;
#20494=DIRECTION ( 'NONE',  ( -0.000000000000000000, -0.000000000000000000, 1.000000000000000000 ) ) ;
#20498=CARTESIAN_POINT ( 'NONE',  ( 45.00000000000000000, -10.00000000000000000, 15.00000000000000000 ) ) ;
#20499=AXIS2_PLACEMENT_3D ( 'NONE', #19442, #9690, #20926 ) ;
#20502=DIRECTION ( 'NONE',  ( -0.000000000000000000, 1.000000000000000000, -0.000000000000000000 ) ) ;
#20513=B_SPLINE_CURVE_WITH_KNOTS ( 'NONE', 3,
 ( #7721, #20445, #4446, #16013, #7823, #4341, #20758, #2756, #1477, #4548, #19179, #6326, #14324, #17487 ),
 .UNSPECIFIED., .F., .F.,
 ( 4, 2, 2, 2, 2, 2, 4 ),
 ( 0.000000000000000000, 0.003003218663418320920, 0.004504827995127496341, 0.006006437326836673064, 0.009009655990255062072, 0.01051126532196427869, 0.01201287465367349358 ),
 .UNSPECIFIED. ) ;
#20524=CARTESIAN_POINT ( 'NONE',  ( -25.16391558800473760, 50.10856639097445253, -14.31252464806517821 ) ) ;
#20528=CARTESIAN_POINT ( 'NONE',  ( -27.76344977743868370, 46.10015299616479467, -4.242667606105982259 ) ) ;
#20534=CARTESIAN_POINT ( 'NONE',  ( -3.197230184752320348, 76.40330993047184904, -2.758159894511169608 ) ) ;
#20538=DIRECTION ( 'NONE',  ( 0.000000000000000000, 0.000000000000000000, 1.000000000000000000 ) ) ;
#20540=CARTESIAN_POINT ( 'NONE',  ( -33.40894099675318074, 52.30484166333695129, -4.500993475257865306 ) ) ;
#20548=CARTESIAN_POINT ( 'NONE',  ( -15.99999999999999289, -9.999999999999994671, 4.999999999999989342 ) ) ;
#20551=EDGE_CURVE ( 'NONE', #4202, #3563, #2006, .T. ) ;
#20555=FACE_OUTER_BOUND ( 'NONE', #16128, .T. ) ;
#20558=CARTESIAN_POINT ( 'NONE',  ( -28.70260728275128415, 67.76582539289573504, 2.255487788205997823 ) ) ;
#20577=CYLINDRICAL_SURFACE ( 'NONE', #5930, 4.999999999999990230 ) ;
#20584=ORIENTED_EDGE ( 'NONE', *, *, #19135, .T. ) ;
#20594=ORIENTED_EDGE ( 'NONE', *, *, #8634, .F. ) ;
#20603=ADVANCED_FACE ( 'NONE', ( #2367 ), #10619, .T. ) ;
#20627=CARTESIAN_POINT ( 'NONE',  ( -8.070106850684350519, 45.02467605610512891, -9.668770963353599868 ) ) ;
#20629=B_SPLINE_CURVE_WITH_KNOTS ( 'NONE', 3,
 ( #13667, #18537, #17054, #18640, #17254, #13987, #4117, #20119, #5581, #4006, #10777, #10455, #2427, #4425, #17153, #10668, #2739, #13874, #8881, #20324, #2638, #1153, #7600, #14092, #20528, #5998, #2946, #17470, #9598, #20940, #14513, #4839, #6517, #4533, #6209, #4938, #17777, #9386, #1254, #9494, #13015, #6103, #11412, #17683, #11002, #17574 ),
 .UNSPECIFIED., .F., .F.,
 ( 4, 2, 2, 2, 2, 2, 2, 2, 2, 2, 2, 2, 2, 2, 2, 2, 2, 2, 2, 2, 2, 2, 4 ),
 ( 0.000000000000000000, 0.002324142326026098875, 0.004648284652052197749, 0.006972426978078296624, 0.009296569304104395498, 0.01162071163013049524, 0.01394485395615659325, 0.01510692511916964312, 0.01626899628218269125, 0.01859313860820877365, 0.01975520977122182179, 0.02091728093423487339, 0.02207935209724792153, 0.02324142326026096966, 0.02556556558628706247, 0.02672763674930011060, 0.02788970791231315527, 0.02905177907532619647, 0.03021385023833924460, 0.03253799256436533394, 0.03370006372737838207, 0.03486213489039143021, 0.03718627721641753342 ),
 .UNSPECIFIED. ) ;
#20632=ORIENTED_EDGE ( 'NONE', *, *, #16814, .F. ) ;
#20636=CARTESIAN_POINT ( 'NONE',  ( -2.552085020148435301, 77.20859777394468892, -3.699063880715907526 ) ) ;
#20641=CARTESIAN_POINT ( 'NONE',  ( -8.315537089352744715, 50.19654607572633154, -14.93280926764117922 ) ) ;
#20656=DIRECTION ( 'NONE',  ( -0.000000000000000000, 1.000000000000000000, -0.000000000000000000 ) ) ;
#20658=ORIENTED_EDGE ( 'NONE', *, *, #4172, .F. ) ;
#20663=ADVANCED_FACE ( 'NONE', ( #12654 ), #17313, .T. ) ;
#20666=VECTOR ( 'NONE', #4647, 1000.000000000000000 ) ;
#20669=CARTESIAN_POINT ( 'NONE',  ( -3.061148255020639919, 72.78546382685976823, 0.3359787457721644111 ) ) ;
#20670=LINE ( 'NONE', #1293, #10343 ) ;
#20677=ORIENTED_EDGE ( 'NONE', *, *, #2807, .T. ) ;
#20678=CARTESIAN_POINT ( 'NONE',  ( 44.00000000000000000, 0.000000000000000000, 15.00000000000000000 ) ) ;
#20683=CARTESIAN_POINT ( 'NONE',  ( 0.05361705196957869402, 61.53954601429751392, 2.100564191518395241 ) ) ;
#20684=AXIS2_PLACEMENT_3D ( 'NONE', #15657, #15760, #14282 ) ;
#20688=ADVANCED_FACE ( 'NONE', ( #2796 ), #2659, .F. ) ;
#20698=AXIS2_PLACEMENT_3D ( 'NONE', #5017, #13098, #12888 ) ;
#20705=ORIENTED_EDGE ( 'NONE', *, *, #20243, .F. ) ;
#20707=DIRECTION ( 'NONE',  ( -1.000000000000000000, -0.000000000000000000, -0.000000000000000000 ) ) ;
#20711=EDGE_CURVE ( 'NONE', #3563, #8008, #434, .T. ) ;
#20725=CIRCLE ( 'NONE', #18692, 12.50000000000000000 ) ;
#20732=CARTESIAN_POINT ( 'NONE',  ( -14.99999999999999645, -9.999999999999998224, 15.00000000000000000 ) ) ;
#20737=AXIS2_PLACEMENT_3D ( 'NONE', #12161, #15257, #5250 ) ;
#20738=CARTESIAN_POINT ( 'NONE',  ( -2.492300918882593308, 50.02397455645809998, -11.50064407951557222 ) ) ;
#20746=CARTESIAN_POINT ( 'NONE',  ( -3.032950703231028555, 76.49637892407336892, -2.857129582000850210 ) ) ;
#20753=CARTESIAN_POINT ( 'NONE',  ( -6.164506467296446246, 50.07147070244224096, -13.99886338058812640 ) ) ;
#20758=CARTESIAN_POINT ( 'NONE',  ( 0.7048535361513451614, 71.96725945621673759, 0.7929198755315660652 ) ) ;
#20775=CARTESIAN_POINT ( 'NONE',  ( -3.273749048447422538, 68.32062926339912678, 2.141136792363729668 ) ) ;
#20781=CARTESIAN_POINT ( 'NONE',  ( -14.99999999999999645, 5.000000000000000000, -30.00000000000000000 ) ) ;
#20783=LINE ( 'NONE', #1404, #196 ) ;
#20796=DIRECTION ( 'NONE',  ( 0.000000000000000000, -1.000000000000000000, 0.000000000000000000 ) ) ;
#20797=CARTESIAN_POINT ( 'NONE',  ( -20.90971454361231352, 15.43716950431552171, 0.9458874751258853353 ) ) ;
#20806=CARTESIAN_POINT ( 'NONE',  ( -32.03950703498303909, 78.52235084885765559, -5.999488569659933823 ) ) ;
#20830=CARTESIAN_POINT ( 'NONE',  ( -3.845968677233049693, 46.83741237530080070, -2.937884555500025474 ) ) ;
#20835=VERTEX_POINT ( 'NONE', #18656 ) ;
#20837=ORIENTED_EDGE ( 'NONE', *, *, #13893, .T. ) ;
#20841=CARTESIAN_POINT ( 'NONE',  ( -7.090779867332545727, 80.00000000007909762, -8.779353540718647153 ) ) ;
#20847=CARTESIAN_POINT ( 'NONE',  ( -31.92009862592069069, 62.68228939152199786, 2.325078759242076298 ) ) ;
#20857=EDGE_CURVE ( 'NONE', #15613, #10630, #2444, .T. ) ;
#20859=CARTESIAN_POINT ( 'NONE',  ( -27.53118063582242669, 59.57781814305143797, 4.826340682015764827 ) ) ;
#20862=CARTESIAN_POINT ( 'NONE',  ( -31.99612686838726461, 68.02992772322291160, 2.199708061508754753 ) ) ;
#20870=FACE_OUTER_BOUND ( 'NONE', #17156, .T. ) ;
#20872=CARTESIAN_POINT ( 'NONE',  ( -29.55702837821359097, 79.40496982188669506, -8.308226455662120813 ) ) ;
#20878=CIRCLE ( 'NONE', #13108, 15.00000000000000000 ) ;
#20889=ORIENTED_EDGE ( 'NONE', *, *, #11234, .T. ) ;
#20895=CARTESIAN_POINT ( 'NONE',  ( -20.90976142674579563, 14.76829926076707089, 0.9456440915044569406 ) ) ;
#20899=ORIENTED_EDGE ( 'NONE', *, *, #8161, .F. ) ;
#20905=CARTESIAN_POINT ( 'NONE',  ( -32.89400105397312046, 77.84073441274443894, -4.744404894156348362 ) ) ;
#20910=AXIS2_PLACEMENT_3D ( 'NONE', #7232, #3953, #17205 ) ;
#20919=VERTEX_POINT ( 'NONE', #9096 ) ;
#20922=CYLINDRICAL_SURFACE ( 'NONE', #8840, 5.999999999999989342 ) ;
#20926=DIRECTION ( 'NONE',  ( 0.000000000000000000, -0.7500000000000006661, -0.6614378277661467909 ) ) ;
#20927=CARTESIAN_POINT ( 'NONE',  ( -26.97244842139108911, 6.114691179184633008, -6.023624517011918478 ) ) ;
#20935=CARTESIAN_POINT ( 'NONE',  ( -9.881800664016866520, 50.28787322564019036, -15.42703672695025752 ) ) ;
#20938=PRODUCT_DEFINITION_FORMATION_WITH_SPECIFIED_SOURCE ( 'ANY', '', #5672, .NOT_KNOWN. ) ;
#20940=CARTESIAN_POINT ( 'NONE',  ( -25.76165165806668611, 45.05596121145901378, -7.817108404872156413 ) ) ;
#20961=COLOUR_RGB('Dark Blue',0.08,0.2,0.34);
#20962=FILL_AREA_STYLE_COLOUR('',#20961);
#20963=FILL_AREA_STYLE('',(#20962));
#20964=SURFACE_STYLE_FILL_AREA(#20963);
#20965=SURFACE_SIDE_STYLE('',(#20964));
#20966=SURFACE_STYLE_USAGE(.BOTH.,#20965);
#20967=PRESENTATION_STYLE_ASSIGNMENT((#20966));
ENDSEC;
END-ISO-10303-21;
